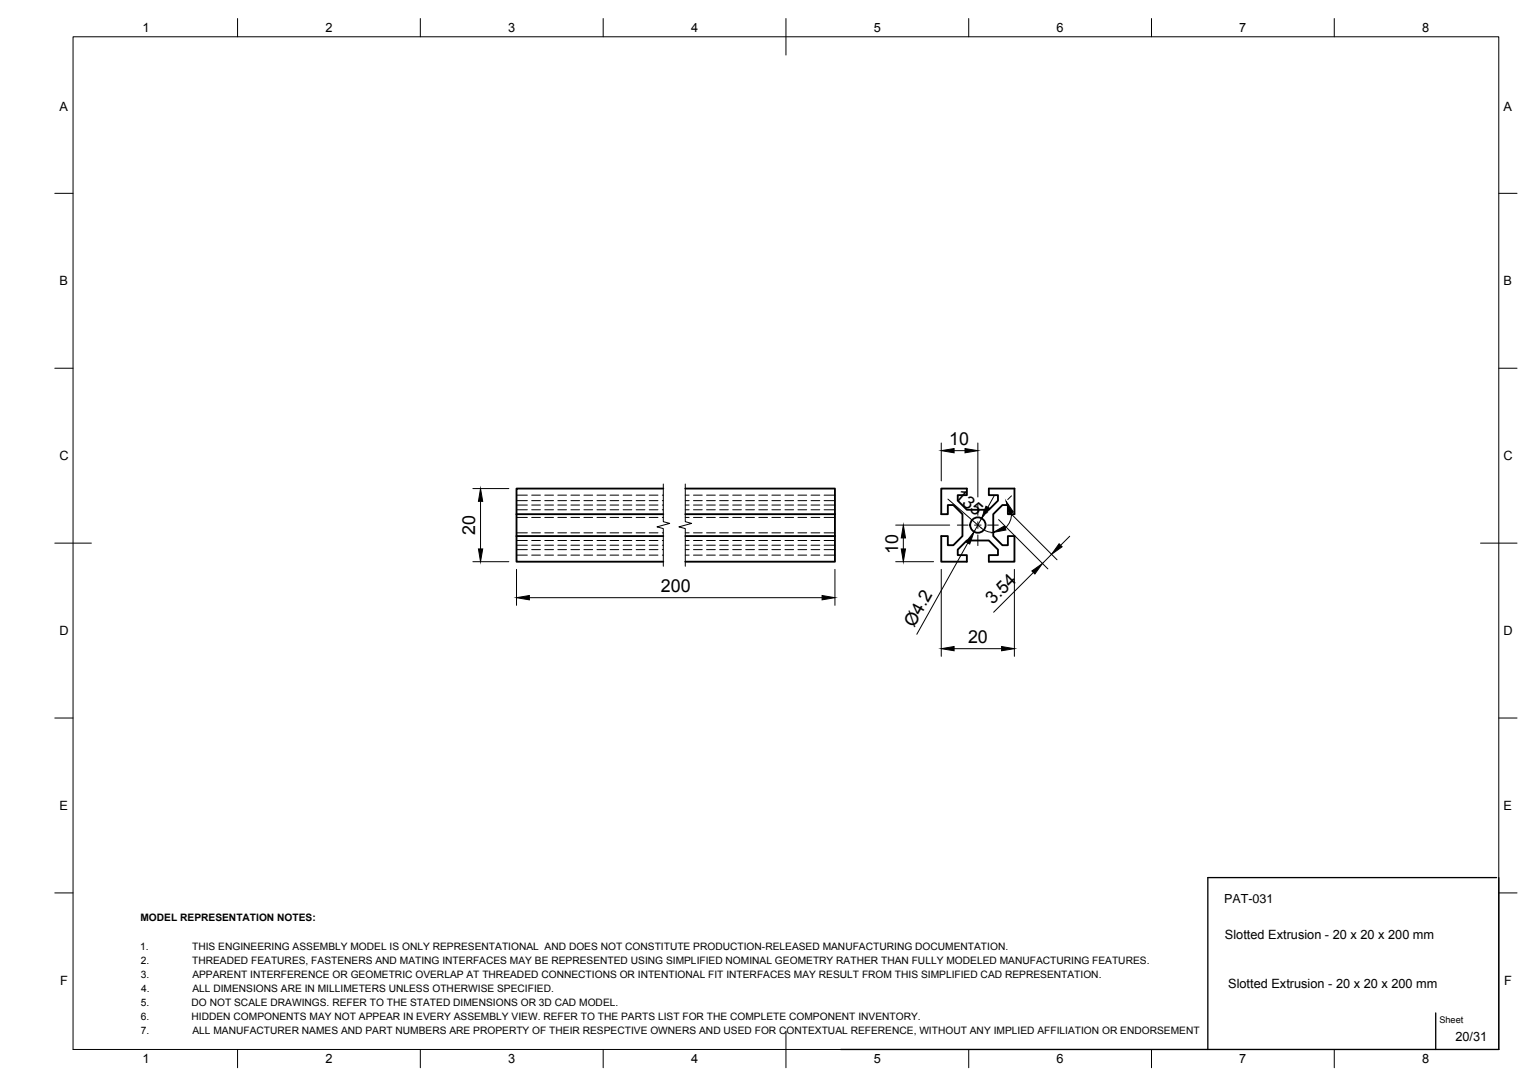
ISO-10303-21;
HEADER;
/* Generated by software containing ST-Developer
 * from STEP Tools, Inc. (www.steptools.com) 
 */

FILE_DESCRIPTION(
/* description */ ('Double-row support with tensioned shaft'),
/* implementation_level */ '2;1');

FILE_NAME(
/* name */ 'Slotted Extrusion - 20 x 20 x 200 mm.step',
/* time_stamp */ '2026-10-27T10:50:35-07:00',
/* author */ (''),
/* organization */ (''),
/* preprocessor_version */ 'ST-DEVELOPER v20.2',
/* originating_system */ 'Autodesk Translation Framework v15.17.0.0',
/* authorisation */ '');

FILE_SCHEMA (('AUTOMOTIVE_DESIGN { 1 0 10303 214 3 1 1 }'));
ENDSEC;

DATA;
#10=MECHANICAL_DESIGN_GEOMETRIC_PRESENTATION_REPRESENTATION('',(#494),#11559);
#430=SHAPE_REPRESENTATION_RELATIONSHIP('SRR','None',#11738,#462);
#462=ADVANCED_BREP_SHAPE_REPRESENTATION('',(#527),#11540);
#494=STYLED_ITEM('',(#11981),#527);
#527=MANIFOLD_SOLID_BREP('Body1',#6339);
#610=FACE_BOUND('',#1479,.T.);
#611=FACE_BOUND('',#1481,.T.);
#741=PLANE('',#6919);
#742=PLANE('',#6920);
#743=PLANE('',#6921);
#744=PLANE('',#6922);
#745=PLANE('',#6923);
#746=PLANE('',#6924);
#747=PLANE('',#6925);
#748=PLANE('',#6926);
#749=PLANE('',#6927);
#750=PLANE('',#6928);
#751=PLANE('',#6929);
#752=PLANE('',#6930);
#753=PLANE('',#6931);
#754=PLANE('',#6932);
#755=PLANE('',#6933);
#756=PLANE('',#6934);
#757=PLANE('',#6935);
#758=PLANE('',#6936);
#759=PLANE('',#6937);
#760=PLANE('',#6938);
#761=PLANE('',#6939);
#762=PLANE('',#6940);
#763=PLANE('',#6941);
#764=PLANE('',#6942);
#765=PLANE('',#6943);
#766=PLANE('',#6944);
#767=PLANE('',#6945);
#768=PLANE('',#6946);
#769=PLANE('',#6947);
#770=PLANE('',#6948);
#771=PLANE('',#6949);
#772=PLANE('',#6950);
#773=PLANE('',#6951);
#774=PLANE('',#6952);
#775=PLANE('',#6953);
#776=PLANE('',#6954);
#777=PLANE('',#6958);
#778=PLANE('',#6959);
#779=PLANE('',#6960);
#780=PLANE('',#6961);
#781=PLANE('',#6962);
#782=PLANE('',#6963);
#783=PLANE('',#6964);
#784=PLANE('',#6965);
#785=PLANE('',#6966);
#786=PLANE('',#6967);
#1021=FACE_OUTER_BOUND('',#1433,.T.);
#1022=FACE_OUTER_BOUND('',#1434,.T.);
#1023=FACE_OUTER_BOUND('',#1435,.T.);
#1024=FACE_OUTER_BOUND('',#1436,.T.);
#1025=FACE_OUTER_BOUND('',#1437,.T.);
#1026=FACE_OUTER_BOUND('',#1438,.T.);
#1027=FACE_OUTER_BOUND('',#1439,.T.);
#1028=FACE_OUTER_BOUND('',#1440,.T.);
#1029=FACE_OUTER_BOUND('',#1441,.T.);
#1030=FACE_OUTER_BOUND('',#1442,.T.);
#1031=FACE_OUTER_BOUND('',#1443,.T.);
#1032=FACE_OUTER_BOUND('',#1444,.T.);
#1033=FACE_OUTER_BOUND('',#1445,.T.);
#1034=FACE_OUTER_BOUND('',#1446,.T.);
#1035=FACE_OUTER_BOUND('',#1447,.T.);
#1036=FACE_OUTER_BOUND('',#1448,.T.);
#1037=FACE_OUTER_BOUND('',#1449,.T.);
#1038=FACE_OUTER_BOUND('',#1450,.T.);
#1039=FACE_OUTER_BOUND('',#1451,.T.);
#1040=FACE_OUTER_BOUND('',#1452,.T.);
#1041=FACE_OUTER_BOUND('',#1453,.T.);
#1042=FACE_OUTER_BOUND('',#1454,.T.);
#1043=FACE_OUTER_BOUND('',#1455,.T.);
#1044=FACE_OUTER_BOUND('',#1456,.T.);
#1045=FACE_OUTER_BOUND('',#1457,.T.);
#1046=FACE_OUTER_BOUND('',#1458,.T.);
#1047=FACE_OUTER_BOUND('',#1459,.T.);
#1048=FACE_OUTER_BOUND('',#1460,.T.);
#1049=FACE_OUTER_BOUND('',#1461,.T.);
#1050=FACE_OUTER_BOUND('',#1462,.T.);
#1051=FACE_OUTER_BOUND('',#1463,.T.);
#1052=FACE_OUTER_BOUND('',#1464,.T.);
#1053=FACE_OUTER_BOUND('',#1465,.T.);
#1054=FACE_OUTER_BOUND('',#1466,.T.);
#1055=FACE_OUTER_BOUND('',#1467,.T.);
#1056=FACE_OUTER_BOUND('',#1468,.T.);
#1057=FACE_OUTER_BOUND('',#1469,.T.);
#1058=FACE_OUTER_BOUND('',#1470,.T.);
#1059=FACE_OUTER_BOUND('',#1471,.T.);
#1060=FACE_OUTER_BOUND('',#1472,.T.);
#1061=FACE_OUTER_BOUND('',#1473,.T.);
#1062=FACE_OUTER_BOUND('',#1474,.T.);
#1063=FACE_OUTER_BOUND('',#1475,.T.);
#1064=FACE_OUTER_BOUND('',#1476,.T.);
#1065=FACE_OUTER_BOUND('',#1477,.T.);
#1066=FACE_OUTER_BOUND('',#1478,.T.);
#1067=FACE_OUTER_BOUND('',#1480,.T.);
#1433=EDGE_LOOP('',(#4774,#4775,#4776,#4777));
#1434=EDGE_LOOP('',(#4778,#4779,#4780,#4781));
#1435=EDGE_LOOP('',(#4782,#4783,#4784,#4785));
#1436=EDGE_LOOP('',(#4786,#4787,#4788,#4789));
#1437=EDGE_LOOP('',(#4790,#4791,#4792,#4793));
#1438=EDGE_LOOP('',(#4794,#4795,#4796,#4797));
#1439=EDGE_LOOP('',(#4798,#4799,#4800,#4801));
#1440=EDGE_LOOP('',(#4802,#4803,#4804,#4805));
#1441=EDGE_LOOP('',(#4806,#4807,#4808,#4809));
#1442=EDGE_LOOP('',(#4810,#4811,#4812,#4813));
#1443=EDGE_LOOP('',(#4814,#4815,#4816,#4817));
#1444=EDGE_LOOP('',(#4818,#4819,#4820,#4821));
#1445=EDGE_LOOP('',(#4822,#4823,#4824,#4825));
#1446=EDGE_LOOP('',(#4826,#4827,#4828,#4829));
#1447=EDGE_LOOP('',(#4830,#4831,#4832,#4833));
#1448=EDGE_LOOP('',(#4834,#4835,#4836,#4837));
#1449=EDGE_LOOP('',(#4838,#4839,#4840,#4841));
#1450=EDGE_LOOP('',(#4842,#4843,#4844,#4845));
#1451=EDGE_LOOP('',(#4846,#4847,#4848,#4849));
#1452=EDGE_LOOP('',(#4850,#4851,#4852,#4853));
#1453=EDGE_LOOP('',(#4854,#4855,#4856,#4857));
#1454=EDGE_LOOP('',(#4858,#4859,#4860,#4861));
#1455=EDGE_LOOP('',(#4862,#4863,#4864,#4865));
#1456=EDGE_LOOP('',(#4866,#4867,#4868,#4869));
#1457=EDGE_LOOP('',(#4870,#4871,#4872,#4873));
#1458=EDGE_LOOP('',(#4874,#4875,#4876,#4877));
#1459=EDGE_LOOP('',(#4878,#4879,#4880,#4881));
#1460=EDGE_LOOP('',(#4882,#4883,#4884,#4885));
#1461=EDGE_LOOP('',(#4886,#4887,#4888,#4889));
#1462=EDGE_LOOP('',(#4890,#4891,#4892,#4893));
#1463=EDGE_LOOP('',(#4894,#4895,#4896,#4897));
#1464=EDGE_LOOP('',(#4898,#4899,#4900,#4901));
#1465=EDGE_LOOP('',(#4902,#4903,#4904,#4905));
#1466=EDGE_LOOP('',(#4906,#4907,#4908,#4909));
#1467=EDGE_LOOP('',(#4910,#4911,#4912,#4913));
#1468=EDGE_LOOP('',(#4914,#4915,#4916,#4917));
#1469=EDGE_LOOP('',(#4918,#4919,#4920,#4921));
#1470=EDGE_LOOP('',(#4922,#4923,#4924,#4925));
#1471=EDGE_LOOP('',(#4926,#4927,#4928,#4929));
#1472=EDGE_LOOP('',(#4930,#4931,#4932,#4933));
#1473=EDGE_LOOP('',(#4934,#4935,#4936,#4937));
#1474=EDGE_LOOP('',(#4938,#4939,#4940,#4941));
#1475=EDGE_LOOP('',(#4942,#4943,#4944,#4945));
#1476=EDGE_LOOP('',(#4946,#4947,#4948,#4949));
#1477=EDGE_LOOP('',(#4950,#4951,#4952,#4953));
#1478=EDGE_LOOP('',(#4954,#4955,#4956,#4957,#4958,#4959,#4960,#4961,#4962,
#4963,#4964,#4965,#4966,#4967,#4968,#4969,#4970,#4971,#4972,#4973,#4974,
#4975,#4976,#4977,#4978,#4979,#4980,#4981,#4982,#4983,#4984,#4985,#4986,
#4987,#4988,#4989,#4990,#4991,#4992,#4993,#4994,#4995,#4996,#4997));
#1479=EDGE_LOOP('',(#4998));
#1480=EDGE_LOOP('',(#4999,#5000,#5001,#5002,#5003,#5004,#5005,#5006,#5007,
#5008,#5009,#5010,#5011,#5012,#5013,#5014,#5015,#5016,#5017,#5018,#5019,
#5020,#5021,#5022,#5023,#5024,#5025,#5026,#5027,#5028,#5029,#5030,#5031,
#5032,#5033,#5034,#5035,#5036,#5037,#5038,#5039,#5040,#5041,#5042));
#1481=EDGE_LOOP('',(#5043));
#1880=LINE('',#9729,#2427);
#1881=LINE('',#9731,#2428);
#1882=LINE('',#9733,#2429);
#1883=LINE('',#9734,#2430);
#1884=LINE('',#9737,#2431);
#1885=LINE('',#9739,#2432);
#1886=LINE('',#9740,#2433);
#1887=LINE('',#9743,#2434);
#1888=LINE('',#9745,#2435);
#1889=LINE('',#9746,#2436);
#1890=LINE('',#9749,#2437);
#1891=LINE('',#9751,#2438);
#1892=LINE('',#9752,#2439);
#1893=LINE('',#9755,#2440);
#1894=LINE('',#9757,#2441);
#1895=LINE('',#9758,#2442);
#1896=LINE('',#9761,#2443);
#1897=LINE('',#9763,#2444);
#1898=LINE('',#9764,#2445);
#1899=LINE('',#9767,#2446);
#1900=LINE('',#9769,#2447);
#1901=LINE('',#9770,#2448);
#1902=LINE('',#9773,#2449);
#1903=LINE('',#9775,#2450);
#1904=LINE('',#9776,#2451);
#1905=LINE('',#9779,#2452);
#1906=LINE('',#9781,#2453);
#1907=LINE('',#9782,#2454);
#1908=LINE('',#9786,#2455);
#1909=LINE('',#9788,#2456);
#1910=LINE('',#9790,#2457);
#1911=LINE('',#9791,#2458);
#1912=LINE('',#9794,#2459);
#1913=LINE('',#9796,#2460);
#1914=LINE('',#9797,#2461);
#1915=LINE('',#9800,#2462);
#1916=LINE('',#9802,#2463);
#1917=LINE('',#9803,#2464);
#1918=LINE('',#9806,#2465);
#1919=LINE('',#9808,#2466);
#1920=LINE('',#9809,#2467);
#1921=LINE('',#9812,#2468);
#1922=LINE('',#9814,#2469);
#1923=LINE('',#9815,#2470);
#1924=LINE('',#9818,#2471);
#1925=LINE('',#9820,#2472);
#1926=LINE('',#9821,#2473);
#1927=LINE('',#9824,#2474);
#1928=LINE('',#9826,#2475);
#1929=LINE('',#9827,#2476);
#1930=LINE('',#9830,#2477);
#1931=LINE('',#9832,#2478);
#1932=LINE('',#9833,#2479);
#1933=LINE('',#9836,#2480);
#1934=LINE('',#9838,#2481);
#1935=LINE('',#9839,#2482);
#1936=LINE('',#9843,#2483);
#1937=LINE('',#9845,#2484);
#1938=LINE('',#9847,#2485);
#1939=LINE('',#9848,#2486);
#1940=LINE('',#9851,#2487);
#1941=LINE('',#9853,#2488);
#1942=LINE('',#9854,#2489);
#1943=LINE('',#9857,#2490);
#1944=LINE('',#9859,#2491);
#1945=LINE('',#9860,#2492);
#1946=LINE('',#9863,#2493);
#1947=LINE('',#9865,#2494);
#1948=LINE('',#9866,#2495);
#1949=LINE('',#9869,#2496);
#1950=LINE('',#9871,#2497);
#1951=LINE('',#9872,#2498);
#1952=LINE('',#9875,#2499);
#1953=LINE('',#9877,#2500);
#1954=LINE('',#9878,#2501);
#1955=LINE('',#9881,#2502);
#1956=LINE('',#9883,#2503);
#1957=LINE('',#9884,#2504);
#1958=LINE('',#9887,#2505);
#1959=LINE('',#9889,#2506);
#1960=LINE('',#9890,#2507);
#1961=LINE('',#9893,#2508);
#1962=LINE('',#9895,#2509);
#1963=LINE('',#9896,#2510);
#1964=LINE('',#9900,#2511);
#1965=LINE('',#9902,#2512);
#1966=LINE('',#9904,#2513);
#1967=LINE('',#9905,#2514);
#1968=LINE('',#9908,#2515);
#1969=LINE('',#9910,#2516);
#1970=LINE('',#9911,#2517);
#1971=LINE('',#9914,#2518);
#1972=LINE('',#9916,#2519);
#1973=LINE('',#9917,#2520);
#1974=LINE('',#9920,#2521);
#1975=LINE('',#9922,#2522);
#1976=LINE('',#9923,#2523);
#1977=LINE('',#9926,#2524);
#1978=LINE('',#9928,#2525);
#1979=LINE('',#9929,#2526);
#1980=LINE('',#9932,#2527);
#1981=LINE('',#9934,#2528);
#1982=LINE('',#9935,#2529);
#1983=LINE('',#9938,#2530);
#1984=LINE('',#9940,#2531);
#1985=LINE('',#9941,#2532);
#1986=LINE('',#9944,#2533);
#1987=LINE('',#9946,#2534);
#1988=LINE('',#9947,#2535);
#1989=LINE('',#9950,#2536);
#1990=LINE('',#9952,#2537);
#1991=LINE('',#9953,#2538);
#1992=LINE('',#9958,#2539);
#1993=LINE('',#9962,#2540);
#1994=LINE('',#9964,#2541);
#1995=LINE('',#9965,#2542);
#1996=LINE('',#9968,#2543);
#1997=LINE('',#9970,#2544);
#1998=LINE('',#9971,#2545);
#1999=LINE('',#9973,#2546);
#2000=LINE('',#9974,#2547);
#2001=LINE('',#9977,#2548);
#2002=LINE('',#9979,#2549);
#2003=LINE('',#9980,#2550);
#2004=LINE('',#9982,#2551);
#2005=LINE('',#9983,#2552);
#2006=LINE('',#9986,#2553);
#2007=LINE('',#9988,#2554);
#2008=LINE('',#9989,#2555);
#2009=LINE('',#9991,#2556);
#2010=LINE('',#9992,#2557);
#2011=LINE('',#9994,#2558);
#2012=LINE('',#9995,#2559);
#2427=VECTOR('',#7923,1.);
#2428=VECTOR('',#7924,1.);
#2429=VECTOR('',#7925,1.);
#2430=VECTOR('',#7926,1.);
#2431=VECTOR('',#7929,1.);
#2432=VECTOR('',#7930,1.);
#2433=VECTOR('',#7931,1.);
#2434=VECTOR('',#7934,1.);
#2435=VECTOR('',#7935,1.);
#2436=VECTOR('',#7936,1.);
#2437=VECTOR('',#7939,1.);
#2438=VECTOR('',#7940,1.);
#2439=VECTOR('',#7941,1.);
#2440=VECTOR('',#7944,1.);
#2441=VECTOR('',#7945,1.);
#2442=VECTOR('',#7946,1.);
#2443=VECTOR('',#7949,1.);
#2444=VECTOR('',#7950,1.);
#2445=VECTOR('',#7951,1.);
#2446=VECTOR('',#7954,1.);
#2447=VECTOR('',#7955,1.);
#2448=VECTOR('',#7956,1.);
#2449=VECTOR('',#7959,1.);
#2450=VECTOR('',#7960,1.);
#2451=VECTOR('',#7961,1.);
#2452=VECTOR('',#7964,1.);
#2453=VECTOR('',#7965,1.);
#2454=VECTOR('',#7966,1.);
#2455=VECTOR('',#7969,1.);
#2456=VECTOR('',#7970,1.);
#2457=VECTOR('',#7971,1.);
#2458=VECTOR('',#7972,1.);
#2459=VECTOR('',#7975,1.);
#2460=VECTOR('',#7976,1.);
#2461=VECTOR('',#7977,1.);
#2462=VECTOR('',#7980,1.);
#2463=VECTOR('',#7981,1.);
#2464=VECTOR('',#7982,1.);
#2465=VECTOR('',#7985,1.);
#2466=VECTOR('',#7986,1.);
#2467=VECTOR('',#7987,1.);
#2468=VECTOR('',#7990,1.);
#2469=VECTOR('',#7991,1.);
#2470=VECTOR('',#7992,1.);
#2471=VECTOR('',#7995,1.);
#2472=VECTOR('',#7996,1.);
#2473=VECTOR('',#7997,1.);
#2474=VECTOR('',#8000,1.);
#2475=VECTOR('',#8001,1.);
#2476=VECTOR('',#8002,1.);
#2477=VECTOR('',#8005,1.);
#2478=VECTOR('',#8006,1.);
#2479=VECTOR('',#8007,1.);
#2480=VECTOR('',#8010,1.);
#2481=VECTOR('',#8011,1.);
#2482=VECTOR('',#8012,1.);
#2483=VECTOR('',#8015,1.);
#2484=VECTOR('',#8016,1.);
#2485=VECTOR('',#8017,1.);
#2486=VECTOR('',#8018,1.);
#2487=VECTOR('',#8021,1.);
#2488=VECTOR('',#8022,1.);
#2489=VECTOR('',#8023,1.);
#2490=VECTOR('',#8026,1.);
#2491=VECTOR('',#8027,1.);
#2492=VECTOR('',#8028,1.);
#2493=VECTOR('',#8031,1.);
#2494=VECTOR('',#8032,1.);
#2495=VECTOR('',#8033,1.);
#2496=VECTOR('',#8036,1.);
#2497=VECTOR('',#8037,1.);
#2498=VECTOR('',#8038,1.);
#2499=VECTOR('',#8041,1.);
#2500=VECTOR('',#8042,1.);
#2501=VECTOR('',#8043,1.);
#2502=VECTOR('',#8046,1.);
#2503=VECTOR('',#8047,1.);
#2504=VECTOR('',#8048,1.);
#2505=VECTOR('',#8051,1.);
#2506=VECTOR('',#8052,1.);
#2507=VECTOR('',#8053,1.);
#2508=VECTOR('',#8056,1.);
#2509=VECTOR('',#8057,1.);
#2510=VECTOR('',#8058,1.);
#2511=VECTOR('',#8061,1.);
#2512=VECTOR('',#8062,1.);
#2513=VECTOR('',#8063,1.);
#2514=VECTOR('',#8064,1.);
#2515=VECTOR('',#8067,1.);
#2516=VECTOR('',#8068,1.);
#2517=VECTOR('',#8069,1.);
#2518=VECTOR('',#8072,1.);
#2519=VECTOR('',#8073,1.);
#2520=VECTOR('',#8074,1.);
#2521=VECTOR('',#8077,1.);
#2522=VECTOR('',#8078,1.);
#2523=VECTOR('',#8079,1.);
#2524=VECTOR('',#8082,1.);
#2525=VECTOR('',#8083,1.);
#2526=VECTOR('',#8084,1.);
#2527=VECTOR('',#8087,1.);
#2528=VECTOR('',#8088,1.);
#2529=VECTOR('',#8089,1.);
#2530=VECTOR('',#8092,1.);
#2531=VECTOR('',#8093,1.);
#2532=VECTOR('',#8094,1.);
#2533=VECTOR('',#8097,1.);
#2534=VECTOR('',#8098,1.);
#2535=VECTOR('',#8099,1.);
#2536=VECTOR('',#8102,1.);
#2537=VECTOR('',#8103,1.);
#2538=VECTOR('',#8104,1.);
#2539=VECTOR('',#8109,0.21);
#2540=VECTOR('',#8114,1.);
#2541=VECTOR('',#8115,1.);
#2542=VECTOR('',#8116,1.);
#2543=VECTOR('',#8119,1.);
#2544=VECTOR('',#8120,1.);
#2545=VECTOR('',#8121,1.);
#2546=VECTOR('',#8124,1.);
#2547=VECTOR('',#8125,1.);
#2548=VECTOR('',#8128,1.);
#2549=VECTOR('',#8129,1.);
#2550=VECTOR('',#8130,1.);
#2551=VECTOR('',#8133,1.);
#2552=VECTOR('',#8134,1.);
#2553=VECTOR('',#8137,1.);
#2554=VECTOR('',#8138,1.);
#2555=VECTOR('',#8139,1.);
#2556=VECTOR('',#8142,1.);
#2557=VECTOR('',#8143,1.);
#2558=VECTOR('',#8146,1.);
#2559=VECTOR('',#8147,1.);
#2920=CIRCLE('',#6956,0.21);
#2921=CIRCLE('',#6957,0.21);
#3175=VERTEX_POINT('',#9727);
#3176=VERTEX_POINT('',#9728);
#3177=VERTEX_POINT('',#9730);
#3178=VERTEX_POINT('',#9732);
#3179=VERTEX_POINT('',#9736);
#3180=VERTEX_POINT('',#9738);
#3181=VERTEX_POINT('',#9742);
#3182=VERTEX_POINT('',#9744);
#3183=VERTEX_POINT('',#9748);
#3184=VERTEX_POINT('',#9750);
#3185=VERTEX_POINT('',#9754);
#3186=VERTEX_POINT('',#9756);
#3187=VERTEX_POINT('',#9760);
#3188=VERTEX_POINT('',#9762);
#3189=VERTEX_POINT('',#9766);
#3190=VERTEX_POINT('',#9768);
#3191=VERTEX_POINT('',#9772);
#3192=VERTEX_POINT('',#9774);
#3193=VERTEX_POINT('',#9778);
#3194=VERTEX_POINT('',#9780);
#3195=VERTEX_POINT('',#9784);
#3196=VERTEX_POINT('',#9785);
#3197=VERTEX_POINT('',#9787);
#3198=VERTEX_POINT('',#9789);
#3199=VERTEX_POINT('',#9793);
#3200=VERTEX_POINT('',#9795);
#3201=VERTEX_POINT('',#9799);
#3202=VERTEX_POINT('',#9801);
#3203=VERTEX_POINT('',#9805);
#3204=VERTEX_POINT('',#9807);
#3205=VERTEX_POINT('',#9811);
#3206=VERTEX_POINT('',#9813);
#3207=VERTEX_POINT('',#9817);
#3208=VERTEX_POINT('',#9819);
#3209=VERTEX_POINT('',#9823);
#3210=VERTEX_POINT('',#9825);
#3211=VERTEX_POINT('',#9829);
#3212=VERTEX_POINT('',#9831);
#3213=VERTEX_POINT('',#9835);
#3214=VERTEX_POINT('',#9837);
#3215=VERTEX_POINT('',#9841);
#3216=VERTEX_POINT('',#9842);
#3217=VERTEX_POINT('',#9844);
#3218=VERTEX_POINT('',#9846);
#3219=VERTEX_POINT('',#9850);
#3220=VERTEX_POINT('',#9852);
#3221=VERTEX_POINT('',#9856);
#3222=VERTEX_POINT('',#9858);
#3223=VERTEX_POINT('',#9862);
#3224=VERTEX_POINT('',#9864);
#3225=VERTEX_POINT('',#9868);
#3226=VERTEX_POINT('',#9870);
#3227=VERTEX_POINT('',#9874);
#3228=VERTEX_POINT('',#9876);
#3229=VERTEX_POINT('',#9880);
#3230=VERTEX_POINT('',#9882);
#3231=VERTEX_POINT('',#9886);
#3232=VERTEX_POINT('',#9888);
#3233=VERTEX_POINT('',#9892);
#3234=VERTEX_POINT('',#9894);
#3235=VERTEX_POINT('',#9898);
#3236=VERTEX_POINT('',#9899);
#3237=VERTEX_POINT('',#9901);
#3238=VERTEX_POINT('',#9903);
#3239=VERTEX_POINT('',#9907);
#3240=VERTEX_POINT('',#9909);
#3241=VERTEX_POINT('',#9913);
#3242=VERTEX_POINT('',#9915);
#3243=VERTEX_POINT('',#9919);
#3244=VERTEX_POINT('',#9921);
#3245=VERTEX_POINT('',#9925);
#3246=VERTEX_POINT('',#9927);
#3247=VERTEX_POINT('',#9931);
#3248=VERTEX_POINT('',#9933);
#3249=VERTEX_POINT('',#9937);
#3250=VERTEX_POINT('',#9939);
#3251=VERTEX_POINT('',#9943);
#3252=VERTEX_POINT('',#9945);
#3253=VERTEX_POINT('',#9949);
#3254=VERTEX_POINT('',#9951);
#3255=VERTEX_POINT('',#9955);
#3256=VERTEX_POINT('',#9957);
#3257=VERTEX_POINT('',#9961);
#3258=VERTEX_POINT('',#9963);
#3259=VERTEX_POINT('',#9967);
#3260=VERTEX_POINT('',#9969);
#3261=VERTEX_POINT('',#9976);
#3262=VERTEX_POINT('',#9978);
#3263=VERTEX_POINT('',#9985);
#3264=VERTEX_POINT('',#9987);
#3772=EDGE_CURVE('',#3175,#3176,#1880,.T.);
#3773=EDGE_CURVE('',#3175,#3177,#1881,.T.);
#3774=EDGE_CURVE('',#3178,#3177,#1882,.T.);
#3775=EDGE_CURVE('',#3176,#3178,#1883,.T.);
#3776=EDGE_CURVE('',#3179,#3175,#1884,.T.);
#3777=EDGE_CURVE('',#3179,#3180,#1885,.T.);
#3778=EDGE_CURVE('',#3177,#3180,#1886,.T.);
#3779=EDGE_CURVE('',#3181,#3179,#1887,.T.);
#3780=EDGE_CURVE('',#3181,#3182,#1888,.T.);
#3781=EDGE_CURVE('',#3180,#3182,#1889,.T.);
#3782=EDGE_CURVE('',#3183,#3181,#1890,.T.);
#3783=EDGE_CURVE('',#3183,#3184,#1891,.T.);
#3784=EDGE_CURVE('',#3182,#3184,#1892,.T.);
#3785=EDGE_CURVE('',#3185,#3183,#1893,.T.);
#3786=EDGE_CURVE('',#3185,#3186,#1894,.T.);
#3787=EDGE_CURVE('',#3184,#3186,#1895,.T.);
#3788=EDGE_CURVE('',#3187,#3185,#1896,.T.);
#3789=EDGE_CURVE('',#3187,#3188,#1897,.T.);
#3790=EDGE_CURVE('',#3186,#3188,#1898,.T.);
#3791=EDGE_CURVE('',#3189,#3187,#1899,.T.);
#3792=EDGE_CURVE('',#3189,#3190,#1900,.T.);
#3793=EDGE_CURVE('',#3188,#3190,#1901,.T.);
#3794=EDGE_CURVE('',#3191,#3189,#1902,.T.);
#3795=EDGE_CURVE('',#3191,#3192,#1903,.T.);
#3796=EDGE_CURVE('',#3190,#3192,#1904,.T.);
#3797=EDGE_CURVE('',#3193,#3191,#1905,.T.);
#3798=EDGE_CURVE('',#3194,#3193,#1906,.T.);
#3799=EDGE_CURVE('',#3192,#3194,#1907,.T.);
#3800=EDGE_CURVE('',#3195,#3196,#1908,.T.);
#3801=EDGE_CURVE('',#3195,#3197,#1909,.T.);
#3802=EDGE_CURVE('',#3198,#3197,#1910,.T.);
#3803=EDGE_CURVE('',#3196,#3198,#1911,.T.);
#3804=EDGE_CURVE('',#3199,#3195,#1912,.T.);
#3805=EDGE_CURVE('',#3199,#3200,#1913,.T.);
#3806=EDGE_CURVE('',#3197,#3200,#1914,.T.);
#3807=EDGE_CURVE('',#3201,#3199,#1915,.T.);
#3808=EDGE_CURVE('',#3201,#3202,#1916,.T.);
#3809=EDGE_CURVE('',#3200,#3202,#1917,.T.);
#3810=EDGE_CURVE('',#3203,#3201,#1918,.T.);
#3811=EDGE_CURVE('',#3203,#3204,#1919,.T.);
#3812=EDGE_CURVE('',#3202,#3204,#1920,.T.);
#3813=EDGE_CURVE('',#3205,#3203,#1921,.T.);
#3814=EDGE_CURVE('',#3205,#3206,#1922,.T.);
#3815=EDGE_CURVE('',#3204,#3206,#1923,.T.);
#3816=EDGE_CURVE('',#3207,#3205,#1924,.T.);
#3817=EDGE_CURVE('',#3207,#3208,#1925,.T.);
#3818=EDGE_CURVE('',#3206,#3208,#1926,.T.);
#3819=EDGE_CURVE('',#3209,#3207,#1927,.T.);
#3820=EDGE_CURVE('',#3209,#3210,#1928,.T.);
#3821=EDGE_CURVE('',#3208,#3210,#1929,.T.);
#3822=EDGE_CURVE('',#3211,#3209,#1930,.T.);
#3823=EDGE_CURVE('',#3211,#3212,#1931,.T.);
#3824=EDGE_CURVE('',#3210,#3212,#1932,.T.);
#3825=EDGE_CURVE('',#3213,#3211,#1933,.T.);
#3826=EDGE_CURVE('',#3214,#3213,#1934,.T.);
#3827=EDGE_CURVE('',#3212,#3214,#1935,.T.);
#3828=EDGE_CURVE('',#3215,#3216,#1936,.T.);
#3829=EDGE_CURVE('',#3215,#3217,#1937,.T.);
#3830=EDGE_CURVE('',#3218,#3217,#1938,.T.);
#3831=EDGE_CURVE('',#3216,#3218,#1939,.T.);
#3832=EDGE_CURVE('',#3219,#3215,#1940,.T.);
#3833=EDGE_CURVE('',#3219,#3220,#1941,.T.);
#3834=EDGE_CURVE('',#3217,#3220,#1942,.T.);
#3835=EDGE_CURVE('',#3221,#3219,#1943,.T.);
#3836=EDGE_CURVE('',#3221,#3222,#1944,.T.);
#3837=EDGE_CURVE('',#3220,#3222,#1945,.T.);
#3838=EDGE_CURVE('',#3223,#3221,#1946,.T.);
#3839=EDGE_CURVE('',#3223,#3224,#1947,.T.);
#3840=EDGE_CURVE('',#3222,#3224,#1948,.T.);
#3841=EDGE_CURVE('',#3225,#3223,#1949,.T.);
#3842=EDGE_CURVE('',#3225,#3226,#1950,.T.);
#3843=EDGE_CURVE('',#3224,#3226,#1951,.T.);
#3844=EDGE_CURVE('',#3227,#3225,#1952,.T.);
#3845=EDGE_CURVE('',#3227,#3228,#1953,.T.);
#3846=EDGE_CURVE('',#3226,#3228,#1954,.T.);
#3847=EDGE_CURVE('',#3229,#3227,#1955,.T.);
#3848=EDGE_CURVE('',#3229,#3230,#1956,.T.);
#3849=EDGE_CURVE('',#3228,#3230,#1957,.T.);
#3850=EDGE_CURVE('',#3231,#3229,#1958,.T.);
#3851=EDGE_CURVE('',#3231,#3232,#1959,.T.);
#3852=EDGE_CURVE('',#3230,#3232,#1960,.T.);
#3853=EDGE_CURVE('',#3233,#3231,#1961,.T.);
#3854=EDGE_CURVE('',#3234,#3233,#1962,.T.);
#3855=EDGE_CURVE('',#3232,#3234,#1963,.T.);
#3856=EDGE_CURVE('',#3235,#3236,#1964,.T.);
#3857=EDGE_CURVE('',#3235,#3237,#1965,.T.);
#3858=EDGE_CURVE('',#3238,#3237,#1966,.T.);
#3859=EDGE_CURVE('',#3236,#3238,#1967,.T.);
#3860=EDGE_CURVE('',#3239,#3235,#1968,.T.);
#3861=EDGE_CURVE('',#3239,#3240,#1969,.T.);
#3862=EDGE_CURVE('',#3237,#3240,#1970,.T.);
#3863=EDGE_CURVE('',#3241,#3239,#1971,.T.);
#3864=EDGE_CURVE('',#3241,#3242,#1972,.T.);
#3865=EDGE_CURVE('',#3240,#3242,#1973,.T.);
#3866=EDGE_CURVE('',#3243,#3241,#1974,.T.);
#3867=EDGE_CURVE('',#3243,#3244,#1975,.T.);
#3868=EDGE_CURVE('',#3242,#3244,#1976,.T.);
#3869=EDGE_CURVE('',#3245,#3243,#1977,.T.);
#3870=EDGE_CURVE('',#3245,#3246,#1978,.T.);
#3871=EDGE_CURVE('',#3244,#3246,#1979,.T.);
#3872=EDGE_CURVE('',#3247,#3245,#1980,.T.);
#3873=EDGE_CURVE('',#3247,#3248,#1981,.T.);
#3874=EDGE_CURVE('',#3246,#3248,#1982,.T.);
#3875=EDGE_CURVE('',#3249,#3247,#1983,.T.);
#3876=EDGE_CURVE('',#3249,#3250,#1984,.T.);
#3877=EDGE_CURVE('',#3248,#3250,#1985,.T.);
#3878=EDGE_CURVE('',#3251,#3249,#1986,.T.);
#3879=EDGE_CURVE('',#3251,#3252,#1987,.T.);
#3880=EDGE_CURVE('',#3250,#3252,#1988,.T.);
#3881=EDGE_CURVE('',#3253,#3251,#1989,.T.);
#3882=EDGE_CURVE('',#3254,#3253,#1990,.T.);
#3883=EDGE_CURVE('',#3252,#3254,#1991,.T.);
#3884=EDGE_CURVE('',#3255,#3255,#2920,.T.);
#3885=EDGE_CURVE('',#3255,#3256,#1992,.T.);
#3886=EDGE_CURVE('',#3256,#3256,#2921,.T.);
#3887=EDGE_CURVE('',#3193,#3257,#1993,.T.);
#3888=EDGE_CURVE('',#3257,#3258,#1994,.T.);
#3889=EDGE_CURVE('',#3194,#3258,#1995,.T.);
#3890=EDGE_CURVE('',#3259,#3178,#1996,.T.);
#3891=EDGE_CURVE('',#3260,#3259,#1997,.T.);
#3892=EDGE_CURVE('',#3260,#3176,#1998,.T.);
#3893=EDGE_CURVE('',#3213,#3260,#1999,.T.);
#3894=EDGE_CURVE('',#3214,#3259,#2000,.T.);
#3895=EDGE_CURVE('',#3261,#3198,#2001,.T.);
#3896=EDGE_CURVE('',#3262,#3261,#2002,.T.);
#3897=EDGE_CURVE('',#3262,#3196,#2003,.T.);
#3898=EDGE_CURVE('',#3233,#3262,#2004,.T.);
#3899=EDGE_CURVE('',#3234,#3261,#2005,.T.);
#3900=EDGE_CURVE('',#3263,#3218,#2006,.T.);
#3901=EDGE_CURVE('',#3264,#3263,#2007,.T.);
#3902=EDGE_CURVE('',#3264,#3216,#2008,.T.);
#3903=EDGE_CURVE('',#3253,#3264,#2009,.T.);
#3904=EDGE_CURVE('',#3254,#3263,#2010,.T.);
#3905=EDGE_CURVE('',#3258,#3238,#2011,.T.);
#3906=EDGE_CURVE('',#3257,#3236,#2012,.T.);
#4774=ORIENTED_EDGE('',*,*,#3772,.F.);
#4775=ORIENTED_EDGE('',*,*,#3773,.T.);
#4776=ORIENTED_EDGE('',*,*,#3774,.F.);
#4777=ORIENTED_EDGE('',*,*,#3775,.F.);
#4778=ORIENTED_EDGE('',*,*,#3776,.F.);
#4779=ORIENTED_EDGE('',*,*,#3777,.T.);
#4780=ORIENTED_EDGE('',*,*,#3778,.F.);
#4781=ORIENTED_EDGE('',*,*,#3773,.F.);
#4782=ORIENTED_EDGE('',*,*,#3779,.F.);
#4783=ORIENTED_EDGE('',*,*,#3780,.T.);
#4784=ORIENTED_EDGE('',*,*,#3781,.F.);
#4785=ORIENTED_EDGE('',*,*,#3777,.F.);
#4786=ORIENTED_EDGE('',*,*,#3782,.F.);
#4787=ORIENTED_EDGE('',*,*,#3783,.T.);
#4788=ORIENTED_EDGE('',*,*,#3784,.F.);
#4789=ORIENTED_EDGE('',*,*,#3780,.F.);
#4790=ORIENTED_EDGE('',*,*,#3785,.F.);
#4791=ORIENTED_EDGE('',*,*,#3786,.T.);
#4792=ORIENTED_EDGE('',*,*,#3787,.F.);
#4793=ORIENTED_EDGE('',*,*,#3783,.F.);
#4794=ORIENTED_EDGE('',*,*,#3788,.F.);
#4795=ORIENTED_EDGE('',*,*,#3789,.T.);
#4796=ORIENTED_EDGE('',*,*,#3790,.F.);
#4797=ORIENTED_EDGE('',*,*,#3786,.F.);
#4798=ORIENTED_EDGE('',*,*,#3791,.F.);
#4799=ORIENTED_EDGE('',*,*,#3792,.T.);
#4800=ORIENTED_EDGE('',*,*,#3793,.F.);
#4801=ORIENTED_EDGE('',*,*,#3789,.F.);
#4802=ORIENTED_EDGE('',*,*,#3794,.F.);
#4803=ORIENTED_EDGE('',*,*,#3795,.T.);
#4804=ORIENTED_EDGE('',*,*,#3796,.F.);
#4805=ORIENTED_EDGE('',*,*,#3792,.F.);
#4806=ORIENTED_EDGE('',*,*,#3797,.F.);
#4807=ORIENTED_EDGE('',*,*,#3798,.F.);
#4808=ORIENTED_EDGE('',*,*,#3799,.F.);
#4809=ORIENTED_EDGE('',*,*,#3795,.F.);
#4810=ORIENTED_EDGE('',*,*,#3800,.F.);
#4811=ORIENTED_EDGE('',*,*,#3801,.T.);
#4812=ORIENTED_EDGE('',*,*,#3802,.F.);
#4813=ORIENTED_EDGE('',*,*,#3803,.F.);
#4814=ORIENTED_EDGE('',*,*,#3804,.F.);
#4815=ORIENTED_EDGE('',*,*,#3805,.T.);
#4816=ORIENTED_EDGE('',*,*,#3806,.F.);
#4817=ORIENTED_EDGE('',*,*,#3801,.F.);
#4818=ORIENTED_EDGE('',*,*,#3807,.F.);
#4819=ORIENTED_EDGE('',*,*,#3808,.T.);
#4820=ORIENTED_EDGE('',*,*,#3809,.F.);
#4821=ORIENTED_EDGE('',*,*,#3805,.F.);
#4822=ORIENTED_EDGE('',*,*,#3810,.F.);
#4823=ORIENTED_EDGE('',*,*,#3811,.T.);
#4824=ORIENTED_EDGE('',*,*,#3812,.F.);
#4825=ORIENTED_EDGE('',*,*,#3808,.F.);
#4826=ORIENTED_EDGE('',*,*,#3813,.F.);
#4827=ORIENTED_EDGE('',*,*,#3814,.T.);
#4828=ORIENTED_EDGE('',*,*,#3815,.F.);
#4829=ORIENTED_EDGE('',*,*,#3811,.F.);
#4830=ORIENTED_EDGE('',*,*,#3816,.F.);
#4831=ORIENTED_EDGE('',*,*,#3817,.T.);
#4832=ORIENTED_EDGE('',*,*,#3818,.F.);
#4833=ORIENTED_EDGE('',*,*,#3814,.F.);
#4834=ORIENTED_EDGE('',*,*,#3819,.F.);
#4835=ORIENTED_EDGE('',*,*,#3820,.T.);
#4836=ORIENTED_EDGE('',*,*,#3821,.F.);
#4837=ORIENTED_EDGE('',*,*,#3817,.F.);
#4838=ORIENTED_EDGE('',*,*,#3822,.F.);
#4839=ORIENTED_EDGE('',*,*,#3823,.T.);
#4840=ORIENTED_EDGE('',*,*,#3824,.F.);
#4841=ORIENTED_EDGE('',*,*,#3820,.F.);
#4842=ORIENTED_EDGE('',*,*,#3825,.F.);
#4843=ORIENTED_EDGE('',*,*,#3826,.F.);
#4844=ORIENTED_EDGE('',*,*,#3827,.F.);
#4845=ORIENTED_EDGE('',*,*,#3823,.F.);
#4846=ORIENTED_EDGE('',*,*,#3828,.F.);
#4847=ORIENTED_EDGE('',*,*,#3829,.T.);
#4848=ORIENTED_EDGE('',*,*,#3830,.F.);
#4849=ORIENTED_EDGE('',*,*,#3831,.F.);
#4850=ORIENTED_EDGE('',*,*,#3832,.F.);
#4851=ORIENTED_EDGE('',*,*,#3833,.T.);
#4852=ORIENTED_EDGE('',*,*,#3834,.F.);
#4853=ORIENTED_EDGE('',*,*,#3829,.F.);
#4854=ORIENTED_EDGE('',*,*,#3835,.F.);
#4855=ORIENTED_EDGE('',*,*,#3836,.T.);
#4856=ORIENTED_EDGE('',*,*,#3837,.F.);
#4857=ORIENTED_EDGE('',*,*,#3833,.F.);
#4858=ORIENTED_EDGE('',*,*,#3838,.F.);
#4859=ORIENTED_EDGE('',*,*,#3839,.T.);
#4860=ORIENTED_EDGE('',*,*,#3840,.F.);
#4861=ORIENTED_EDGE('',*,*,#3836,.F.);
#4862=ORIENTED_EDGE('',*,*,#3841,.F.);
#4863=ORIENTED_EDGE('',*,*,#3842,.T.);
#4864=ORIENTED_EDGE('',*,*,#3843,.F.);
#4865=ORIENTED_EDGE('',*,*,#3839,.F.);
#4866=ORIENTED_EDGE('',*,*,#3844,.F.);
#4867=ORIENTED_EDGE('',*,*,#3845,.T.);
#4868=ORIENTED_EDGE('',*,*,#3846,.F.);
#4869=ORIENTED_EDGE('',*,*,#3842,.F.);
#4870=ORIENTED_EDGE('',*,*,#3847,.F.);
#4871=ORIENTED_EDGE('',*,*,#3848,.T.);
#4872=ORIENTED_EDGE('',*,*,#3849,.F.);
#4873=ORIENTED_EDGE('',*,*,#3845,.F.);
#4874=ORIENTED_EDGE('',*,*,#3850,.F.);
#4875=ORIENTED_EDGE('',*,*,#3851,.T.);
#4876=ORIENTED_EDGE('',*,*,#3852,.F.);
#4877=ORIENTED_EDGE('',*,*,#3848,.F.);
#4878=ORIENTED_EDGE('',*,*,#3853,.F.);
#4879=ORIENTED_EDGE('',*,*,#3854,.F.);
#4880=ORIENTED_EDGE('',*,*,#3855,.F.);
#4881=ORIENTED_EDGE('',*,*,#3851,.F.);
#4882=ORIENTED_EDGE('',*,*,#3856,.F.);
#4883=ORIENTED_EDGE('',*,*,#3857,.T.);
#4884=ORIENTED_EDGE('',*,*,#3858,.F.);
#4885=ORIENTED_EDGE('',*,*,#3859,.F.);
#4886=ORIENTED_EDGE('',*,*,#3860,.F.);
#4887=ORIENTED_EDGE('',*,*,#3861,.T.);
#4888=ORIENTED_EDGE('',*,*,#3862,.F.);
#4889=ORIENTED_EDGE('',*,*,#3857,.F.);
#4890=ORIENTED_EDGE('',*,*,#3863,.F.);
#4891=ORIENTED_EDGE('',*,*,#3864,.T.);
#4892=ORIENTED_EDGE('',*,*,#3865,.F.);
#4893=ORIENTED_EDGE('',*,*,#3861,.F.);
#4894=ORIENTED_EDGE('',*,*,#3866,.F.);
#4895=ORIENTED_EDGE('',*,*,#3867,.T.);
#4896=ORIENTED_EDGE('',*,*,#3868,.F.);
#4897=ORIENTED_EDGE('',*,*,#3864,.F.);
#4898=ORIENTED_EDGE('',*,*,#3869,.F.);
#4899=ORIENTED_EDGE('',*,*,#3870,.T.);
#4900=ORIENTED_EDGE('',*,*,#3871,.F.);
#4901=ORIENTED_EDGE('',*,*,#3867,.F.);
#4902=ORIENTED_EDGE('',*,*,#3872,.F.);
#4903=ORIENTED_EDGE('',*,*,#3873,.T.);
#4904=ORIENTED_EDGE('',*,*,#3874,.F.);
#4905=ORIENTED_EDGE('',*,*,#3870,.F.);
#4906=ORIENTED_EDGE('',*,*,#3875,.F.);
#4907=ORIENTED_EDGE('',*,*,#3876,.T.);
#4908=ORIENTED_EDGE('',*,*,#3877,.F.);
#4909=ORIENTED_EDGE('',*,*,#3873,.F.);
#4910=ORIENTED_EDGE('',*,*,#3878,.F.);
#4911=ORIENTED_EDGE('',*,*,#3879,.T.);
#4912=ORIENTED_EDGE('',*,*,#3880,.F.);
#4913=ORIENTED_EDGE('',*,*,#3876,.F.);
#4914=ORIENTED_EDGE('',*,*,#3881,.F.);
#4915=ORIENTED_EDGE('',*,*,#3882,.F.);
#4916=ORIENTED_EDGE('',*,*,#3883,.F.);
#4917=ORIENTED_EDGE('',*,*,#3879,.F.);
#4918=ORIENTED_EDGE('',*,*,#3884,.F.);
#4919=ORIENTED_EDGE('',*,*,#3885,.T.);
#4920=ORIENTED_EDGE('',*,*,#3886,.F.);
#4921=ORIENTED_EDGE('',*,*,#3885,.F.);
#4922=ORIENTED_EDGE('',*,*,#3798,.T.);
#4923=ORIENTED_EDGE('',*,*,#3887,.T.);
#4924=ORIENTED_EDGE('',*,*,#3888,.T.);
#4925=ORIENTED_EDGE('',*,*,#3889,.F.);
#4926=ORIENTED_EDGE('',*,*,#3775,.T.);
#4927=ORIENTED_EDGE('',*,*,#3890,.F.);
#4928=ORIENTED_EDGE('',*,*,#3891,.F.);
#4929=ORIENTED_EDGE('',*,*,#3892,.T.);
#4930=ORIENTED_EDGE('',*,*,#3826,.T.);
#4931=ORIENTED_EDGE('',*,*,#3893,.T.);
#4932=ORIENTED_EDGE('',*,*,#3891,.T.);
#4933=ORIENTED_EDGE('',*,*,#3894,.F.);
#4934=ORIENTED_EDGE('',*,*,#3803,.T.);
#4935=ORIENTED_EDGE('',*,*,#3895,.F.);
#4936=ORIENTED_EDGE('',*,*,#3896,.F.);
#4937=ORIENTED_EDGE('',*,*,#3897,.T.);
#4938=ORIENTED_EDGE('',*,*,#3854,.T.);
#4939=ORIENTED_EDGE('',*,*,#3898,.T.);
#4940=ORIENTED_EDGE('',*,*,#3896,.T.);
#4941=ORIENTED_EDGE('',*,*,#3899,.F.);
#4942=ORIENTED_EDGE('',*,*,#3831,.T.);
#4943=ORIENTED_EDGE('',*,*,#3900,.F.);
#4944=ORIENTED_EDGE('',*,*,#3901,.F.);
#4945=ORIENTED_EDGE('',*,*,#3902,.T.);
#4946=ORIENTED_EDGE('',*,*,#3882,.T.);
#4947=ORIENTED_EDGE('',*,*,#3903,.T.);
#4948=ORIENTED_EDGE('',*,*,#3901,.T.);
#4949=ORIENTED_EDGE('',*,*,#3904,.F.);
#4950=ORIENTED_EDGE('',*,*,#3859,.T.);
#4951=ORIENTED_EDGE('',*,*,#3905,.F.);
#4952=ORIENTED_EDGE('',*,*,#3888,.F.);
#4953=ORIENTED_EDGE('',*,*,#3906,.T.);
#4954=ORIENTED_EDGE('',*,*,#3774,.T.);
#4955=ORIENTED_EDGE('',*,*,#3778,.T.);
#4956=ORIENTED_EDGE('',*,*,#3781,.T.);
#4957=ORIENTED_EDGE('',*,*,#3784,.T.);
#4958=ORIENTED_EDGE('',*,*,#3787,.T.);
#4959=ORIENTED_EDGE('',*,*,#3790,.T.);
#4960=ORIENTED_EDGE('',*,*,#3793,.T.);
#4961=ORIENTED_EDGE('',*,*,#3796,.T.);
#4962=ORIENTED_EDGE('',*,*,#3799,.T.);
#4963=ORIENTED_EDGE('',*,*,#3889,.T.);
#4964=ORIENTED_EDGE('',*,*,#3905,.T.);
#4965=ORIENTED_EDGE('',*,*,#3858,.T.);
#4966=ORIENTED_EDGE('',*,*,#3862,.T.);
#4967=ORIENTED_EDGE('',*,*,#3865,.T.);
#4968=ORIENTED_EDGE('',*,*,#3868,.T.);
#4969=ORIENTED_EDGE('',*,*,#3871,.T.);
#4970=ORIENTED_EDGE('',*,*,#3874,.T.);
#4971=ORIENTED_EDGE('',*,*,#3877,.T.);
#4972=ORIENTED_EDGE('',*,*,#3880,.T.);
#4973=ORIENTED_EDGE('',*,*,#3883,.T.);
#4974=ORIENTED_EDGE('',*,*,#3904,.T.);
#4975=ORIENTED_EDGE('',*,*,#3900,.T.);
#4976=ORIENTED_EDGE('',*,*,#3830,.T.);
#4977=ORIENTED_EDGE('',*,*,#3834,.T.);
#4978=ORIENTED_EDGE('',*,*,#3837,.T.);
#4979=ORIENTED_EDGE('',*,*,#3840,.T.);
#4980=ORIENTED_EDGE('',*,*,#3843,.T.);
#4981=ORIENTED_EDGE('',*,*,#3846,.T.);
#4982=ORIENTED_EDGE('',*,*,#3849,.T.);
#4983=ORIENTED_EDGE('',*,*,#3852,.T.);
#4984=ORIENTED_EDGE('',*,*,#3855,.T.);
#4985=ORIENTED_EDGE('',*,*,#3899,.T.);
#4986=ORIENTED_EDGE('',*,*,#3895,.T.);
#4987=ORIENTED_EDGE('',*,*,#3802,.T.);
#4988=ORIENTED_EDGE('',*,*,#3806,.T.);
#4989=ORIENTED_EDGE('',*,*,#3809,.T.);
#4990=ORIENTED_EDGE('',*,*,#3812,.T.);
#4991=ORIENTED_EDGE('',*,*,#3815,.T.);
#4992=ORIENTED_EDGE('',*,*,#3818,.T.);
#4993=ORIENTED_EDGE('',*,*,#3821,.T.);
#4994=ORIENTED_EDGE('',*,*,#3824,.T.);
#4995=ORIENTED_EDGE('',*,*,#3827,.T.);
#4996=ORIENTED_EDGE('',*,*,#3894,.T.);
#4997=ORIENTED_EDGE('',*,*,#3890,.T.);
#4998=ORIENTED_EDGE('',*,*,#3886,.T.);
#4999=ORIENTED_EDGE('',*,*,#3772,.T.);
#5000=ORIENTED_EDGE('',*,*,#3892,.F.);
#5001=ORIENTED_EDGE('',*,*,#3893,.F.);
#5002=ORIENTED_EDGE('',*,*,#3825,.T.);
#5003=ORIENTED_EDGE('',*,*,#3822,.T.);
#5004=ORIENTED_EDGE('',*,*,#3819,.T.);
#5005=ORIENTED_EDGE('',*,*,#3816,.T.);
#5006=ORIENTED_EDGE('',*,*,#3813,.T.);
#5007=ORIENTED_EDGE('',*,*,#3810,.T.);
#5008=ORIENTED_EDGE('',*,*,#3807,.T.);
#5009=ORIENTED_EDGE('',*,*,#3804,.T.);
#5010=ORIENTED_EDGE('',*,*,#3800,.T.);
#5011=ORIENTED_EDGE('',*,*,#3897,.F.);
#5012=ORIENTED_EDGE('',*,*,#3898,.F.);
#5013=ORIENTED_EDGE('',*,*,#3853,.T.);
#5014=ORIENTED_EDGE('',*,*,#3850,.T.);
#5015=ORIENTED_EDGE('',*,*,#3847,.T.);
#5016=ORIENTED_EDGE('',*,*,#3844,.T.);
#5017=ORIENTED_EDGE('',*,*,#3841,.T.);
#5018=ORIENTED_EDGE('',*,*,#3838,.T.);
#5019=ORIENTED_EDGE('',*,*,#3835,.T.);
#5020=ORIENTED_EDGE('',*,*,#3832,.T.);
#5021=ORIENTED_EDGE('',*,*,#3828,.T.);
#5022=ORIENTED_EDGE('',*,*,#3902,.F.);
#5023=ORIENTED_EDGE('',*,*,#3903,.F.);
#5024=ORIENTED_EDGE('',*,*,#3881,.T.);
#5025=ORIENTED_EDGE('',*,*,#3878,.T.);
#5026=ORIENTED_EDGE('',*,*,#3875,.T.);
#5027=ORIENTED_EDGE('',*,*,#3872,.T.);
#5028=ORIENTED_EDGE('',*,*,#3869,.T.);
#5029=ORIENTED_EDGE('',*,*,#3866,.T.);
#5030=ORIENTED_EDGE('',*,*,#3863,.T.);
#5031=ORIENTED_EDGE('',*,*,#3860,.T.);
#5032=ORIENTED_EDGE('',*,*,#3856,.T.);
#5033=ORIENTED_EDGE('',*,*,#3906,.F.);
#5034=ORIENTED_EDGE('',*,*,#3887,.F.);
#5035=ORIENTED_EDGE('',*,*,#3797,.T.);
#5036=ORIENTED_EDGE('',*,*,#3794,.T.);
#5037=ORIENTED_EDGE('',*,*,#3791,.T.);
#5038=ORIENTED_EDGE('',*,*,#3788,.T.);
#5039=ORIENTED_EDGE('',*,*,#3785,.T.);
#5040=ORIENTED_EDGE('',*,*,#3782,.T.);
#5041=ORIENTED_EDGE('',*,*,#3779,.T.);
#5042=ORIENTED_EDGE('',*,*,#3776,.T.);
#5043=ORIENTED_EDGE('',*,*,#3884,.T.);
#5932=CYLINDRICAL_SURFACE('',#6955,0.21);
#6084=ADVANCED_FACE('',(#1021),#741,.F.);
#6085=ADVANCED_FACE('',(#1022),#742,.F.);
#6086=ADVANCED_FACE('',(#1023),#743,.F.);
#6087=ADVANCED_FACE('',(#1024),#744,.F.);
#6088=ADVANCED_FACE('',(#1025),#745,.F.);
#6089=ADVANCED_FACE('',(#1026),#746,.F.);
#6090=ADVANCED_FACE('',(#1027),#747,.F.);
#6091=ADVANCED_FACE('',(#1028),#748,.F.);
#6092=ADVANCED_FACE('',(#1029),#749,.F.);
#6093=ADVANCED_FACE('',(#1030),#750,.F.);
#6094=ADVANCED_FACE('',(#1031),#751,.F.);
#6095=ADVANCED_FACE('',(#1032),#752,.F.);
#6096=ADVANCED_FACE('',(#1033),#753,.F.);
#6097=ADVANCED_FACE('',(#1034),#754,.F.);
#6098=ADVANCED_FACE('',(#1035),#755,.F.);
#6099=ADVANCED_FACE('',(#1036),#756,.F.);
#6100=ADVANCED_FACE('',(#1037),#757,.F.);
#6101=ADVANCED_FACE('',(#1038),#758,.F.);
#6102=ADVANCED_FACE('',(#1039),#759,.F.);
#6103=ADVANCED_FACE('',(#1040),#760,.F.);
#6104=ADVANCED_FACE('',(#1041),#761,.F.);
#6105=ADVANCED_FACE('',(#1042),#762,.F.);
#6106=ADVANCED_FACE('',(#1043),#763,.F.);
#6107=ADVANCED_FACE('',(#1044),#764,.F.);
#6108=ADVANCED_FACE('',(#1045),#765,.F.);
#6109=ADVANCED_FACE('',(#1046),#766,.F.);
#6110=ADVANCED_FACE('',(#1047),#767,.F.);
#6111=ADVANCED_FACE('',(#1048),#768,.F.);
#6112=ADVANCED_FACE('',(#1049),#769,.F.);
#6113=ADVANCED_FACE('',(#1050),#770,.F.);
#6114=ADVANCED_FACE('',(#1051),#771,.F.);
#6115=ADVANCED_FACE('',(#1052),#772,.F.);
#6116=ADVANCED_FACE('',(#1053),#773,.F.);
#6117=ADVANCED_FACE('',(#1054),#774,.F.);
#6118=ADVANCED_FACE('',(#1055),#775,.F.);
#6119=ADVANCED_FACE('',(#1056),#776,.F.);
#6120=ADVANCED_FACE('',(#1057),#5932,.F.);
#6121=ADVANCED_FACE('',(#1058),#777,.T.);
#6122=ADVANCED_FACE('',(#1059),#778,.T.);
#6123=ADVANCED_FACE('',(#1060),#779,.T.);
#6124=ADVANCED_FACE('',(#1061),#780,.T.);
#6125=ADVANCED_FACE('',(#1062),#781,.T.);
#6126=ADVANCED_FACE('',(#1063),#782,.T.);
#6127=ADVANCED_FACE('',(#1064),#783,.T.);
#6128=ADVANCED_FACE('',(#1065),#784,.T.);
#6129=ADVANCED_FACE('',(#1066,#610),#785,.T.);
#6130=ADVANCED_FACE('',(#1067,#611),#786,.F.);
#6339=CLOSED_SHELL('',(#6084,#6085,#6086,#6087,#6088,#6089,#6090,#6091,
#6092,#6093,#6094,#6095,#6096,#6097,#6098,#6099,#6100,#6101,#6102,#6103,
#6104,#6105,#6106,#6107,#6108,#6109,#6110,#6111,#6112,#6113,#6114,#6115,
#6116,#6117,#6118,#6119,#6120,#6121,#6122,#6123,#6124,#6125,#6126,#6127,
#6128,#6129,#6130));
#6918=AXIS2_PLACEMENT_3D('',#9725,#7919,#7920);
#6919=AXIS2_PLACEMENT_3D('',#9726,#7921,#7922);
#6920=AXIS2_PLACEMENT_3D('',#9735,#7927,#7928);
#6921=AXIS2_PLACEMENT_3D('',#9741,#7932,#7933);
#6922=AXIS2_PLACEMENT_3D('',#9747,#7937,#7938);
#6923=AXIS2_PLACEMENT_3D('',#9753,#7942,#7943);
#6924=AXIS2_PLACEMENT_3D('',#9759,#7947,#7948);
#6925=AXIS2_PLACEMENT_3D('',#9765,#7952,#7953);
#6926=AXIS2_PLACEMENT_3D('',#9771,#7957,#7958);
#6927=AXIS2_PLACEMENT_3D('',#9777,#7962,#7963);
#6928=AXIS2_PLACEMENT_3D('',#9783,#7967,#7968);
#6929=AXIS2_PLACEMENT_3D('',#9792,#7973,#7974);
#6930=AXIS2_PLACEMENT_3D('',#9798,#7978,#7979);
#6931=AXIS2_PLACEMENT_3D('',#9804,#7983,#7984);
#6932=AXIS2_PLACEMENT_3D('',#9810,#7988,#7989);
#6933=AXIS2_PLACEMENT_3D('',#9816,#7993,#7994);
#6934=AXIS2_PLACEMENT_3D('',#9822,#7998,#7999);
#6935=AXIS2_PLACEMENT_3D('',#9828,#8003,#8004);
#6936=AXIS2_PLACEMENT_3D('',#9834,#8008,#8009);
#6937=AXIS2_PLACEMENT_3D('',#9840,#8013,#8014);
#6938=AXIS2_PLACEMENT_3D('',#9849,#8019,#8020);
#6939=AXIS2_PLACEMENT_3D('',#9855,#8024,#8025);
#6940=AXIS2_PLACEMENT_3D('',#9861,#8029,#8030);
#6941=AXIS2_PLACEMENT_3D('',#9867,#8034,#8035);
#6942=AXIS2_PLACEMENT_3D('',#9873,#8039,#8040);
#6943=AXIS2_PLACEMENT_3D('',#9879,#8044,#8045);
#6944=AXIS2_PLACEMENT_3D('',#9885,#8049,#8050);
#6945=AXIS2_PLACEMENT_3D('',#9891,#8054,#8055);
#6946=AXIS2_PLACEMENT_3D('',#9897,#8059,#8060);
#6947=AXIS2_PLACEMENT_3D('',#9906,#8065,#8066);
#6948=AXIS2_PLACEMENT_3D('',#9912,#8070,#8071);
#6949=AXIS2_PLACEMENT_3D('',#9918,#8075,#8076);
#6950=AXIS2_PLACEMENT_3D('',#9924,#8080,#8081);
#6951=AXIS2_PLACEMENT_3D('',#9930,#8085,#8086);
#6952=AXIS2_PLACEMENT_3D('',#9936,#8090,#8091);
#6953=AXIS2_PLACEMENT_3D('',#9942,#8095,#8096);
#6954=AXIS2_PLACEMENT_3D('',#9948,#8100,#8101);
#6955=AXIS2_PLACEMENT_3D('',#9954,#8105,#8106);
#6956=AXIS2_PLACEMENT_3D('',#9956,#8107,#8108);
#6957=AXIS2_PLACEMENT_3D('',#9959,#8110,#8111);
#6958=AXIS2_PLACEMENT_3D('',#9960,#8112,#8113);
#6959=AXIS2_PLACEMENT_3D('',#9966,#8117,#8118);
#6960=AXIS2_PLACEMENT_3D('',#9972,#8122,#8123);
#6961=AXIS2_PLACEMENT_3D('',#9975,#8126,#8127);
#6962=AXIS2_PLACEMENT_3D('',#9981,#8131,#8132);
#6963=AXIS2_PLACEMENT_3D('',#9984,#8135,#8136);
#6964=AXIS2_PLACEMENT_3D('',#9990,#8140,#8141);
#6965=AXIS2_PLACEMENT_3D('',#9993,#8144,#8145);
#6966=AXIS2_PLACEMENT_3D('',#9996,#8148,#8149);
#6967=AXIS2_PLACEMENT_3D('',#9997,#8150,#8151);
#7919=DIRECTION('axis',(0.,0.,1.));
#7920=DIRECTION('refdir',(1.,0.,0.));
#7921=DIRECTION('center_axis',(0.,0.,-1.));
#7922=DIRECTION('ref_axis',(0.,1.,0.));
#7923=DIRECTION('',(0.,1.,0.));
#7924=DIRECTION('',(1.,0.,0.));
#7925=DIRECTION('',(0.,-1.,0.));
#7926=DIRECTION('',(1.,0.,0.));
#7927=DIRECTION('center_axis',(0.,1.,-8.88178419700125E-16));
#7928=DIRECTION('ref_axis',(0.,8.88178419700125E-16,1.));
#7929=DIRECTION('',(0.,8.88178419700125E-16,1.));
#7930=DIRECTION('',(1.,0.,0.));
#7931=DIRECTION('',(0.,-8.88178419700125E-16,-1.));
#7932=DIRECTION('center_axis',(0.,-7.40148683083439E-16,-1.));
#7933=DIRECTION('ref_axis',(0.,1.,-7.40148683083439E-16));
#7934=DIRECTION('',(0.,1.,-7.40148683083439E-16));
#7935=DIRECTION('',(1.,0.,0.));
#7936=DIRECTION('',(0.,-1.,7.40148683083439E-16));
#7937=DIRECTION('center_axis',(0.,-0.707106781186547,-0.707106781186548));
#7938=DIRECTION('ref_axis',(0.,0.707106781186548,-0.707106781186547));
#7939=DIRECTION('',(0.,0.707106781186548,-0.707106781186547));
#7940=DIRECTION('',(1.,0.,0.));
#7941=DIRECTION('',(0.,-0.707106781186548,0.707106781186547));
#7942=DIRECTION('center_axis',(0.,-1.,2.77555756156289E-16));
#7943=DIRECTION('ref_axis',(0.,-2.77555756156289E-16,-1.));
#7944=DIRECTION('',(0.,-2.77555756156289E-16,-1.));
#7945=DIRECTION('',(1.,0.,0.));
#7946=DIRECTION('',(0.,2.77555756156289E-16,1.));
#7947=DIRECTION('center_axis',(0.,-0.707106781186547,0.707106781186548));
#7948=DIRECTION('ref_axis',(0.,-0.707106781186548,-0.707106781186547));
#7949=DIRECTION('',(0.,-0.707106781186548,-0.707106781186547));
#7950=DIRECTION('',(1.,0.,0.));
#7951=DIRECTION('',(0.,0.707106781186548,0.707106781186547));
#7952=DIRECTION('center_axis',(0.,7.40148683083438E-16,1.));
#7953=DIRECTION('ref_axis',(0.,-1.,7.40148683083438E-16));
#7954=DIRECTION('',(0.,-1.,7.40148683083438E-16));
#7955=DIRECTION('',(1.,0.,0.));
#7956=DIRECTION('',(0.,1.,-7.40148683083438E-16));
#7957=DIRECTION('center_axis',(0.,1.,-4.44089209850063E-16));
#7958=DIRECTION('ref_axis',(0.,4.44089209850063E-16,1.));
#7959=DIRECTION('',(0.,4.44089209850063E-16,1.));
#7960=DIRECTION('',(1.,0.,0.));
#7961=DIRECTION('',(0.,-4.44089209850063E-16,-1.));
#7962=DIRECTION('center_axis',(0.,2.41352831440251E-16,1.));
#7963=DIRECTION('ref_axis',(0.,-1.,2.41352831440251E-16));
#7964=DIRECTION('',(0.,-1.,2.41352831440251E-16));
#7965=DIRECTION('',(-1.,0.,0.));
#7966=DIRECTION('',(0.,1.,-2.41352831440251E-16));
#7967=DIRECTION('center_axis',(0.,-1.,2.41352831440251E-16));
#7968=DIRECTION('ref_axis',(0.,-2.41352831440251E-16,-1.));
#7969=DIRECTION('',(0.,-2.41352831440251E-16,-1.));
#7970=DIRECTION('',(1.,0.,0.));
#7971=DIRECTION('',(0.,2.41352831440251E-16,1.));
#7972=DIRECTION('',(1.,0.,0.));
#7973=DIRECTION('center_axis',(0.,0.,-1.));
#7974=DIRECTION('ref_axis',(0.,1.,0.));
#7975=DIRECTION('',(0.,1.,0.));
#7976=DIRECTION('',(1.,0.,0.));
#7977=DIRECTION('',(0.,-1.,0.));
#7978=DIRECTION('center_axis',(0.,-1.,0.));
#7979=DIRECTION('ref_axis',(0.,0.,-1.));
#7980=DIRECTION('',(0.,0.,-1.));
#7981=DIRECTION('',(1.,0.,0.));
#7982=DIRECTION('',(0.,0.,1.));
#7983=DIRECTION('center_axis',(0.,-0.707106781186547,0.707106781186548));
#7984=DIRECTION('ref_axis',(0.,-0.707106781186548,-0.707106781186547));
#7985=DIRECTION('',(0.,-0.707106781186548,-0.707106781186547));
#7986=DIRECTION('',(1.,0.,0.));
#7987=DIRECTION('',(0.,0.707106781186548,0.707106781186547));
#7988=DIRECTION('center_axis',(0.,0.,1.));
#7989=DIRECTION('ref_axis',(0.,-1.,0.));
#7990=DIRECTION('',(0.,-1.,0.));
#7991=DIRECTION('',(1.,0.,0.));
#7992=DIRECTION('',(0.,1.,0.));
#7993=DIRECTION('center_axis',(0.,0.707106781186548,0.707106781186547));
#7994=DIRECTION('ref_axis',(0.,-0.707106781186547,0.707106781186548));
#7995=DIRECTION('',(0.,-0.707106781186547,0.707106781186548));
#7996=DIRECTION('',(1.,0.,0.));
#7997=DIRECTION('',(0.,0.707106781186547,-0.707106781186548));
#7998=DIRECTION('center_axis',(0.,1.,0.));
#7999=DIRECTION('ref_axis',(0.,0.,1.));
#8000=DIRECTION('',(0.,0.,1.));
#8001=DIRECTION('',(1.,0.,0.));
#8002=DIRECTION('',(0.,0.,-1.));
#8003=DIRECTION('center_axis',(0.,0.,-1.));
#8004=DIRECTION('ref_axis',(0.,1.,0.));
#8005=DIRECTION('',(0.,1.,0.));
#8006=DIRECTION('',(1.,0.,0.));
#8007=DIRECTION('',(0.,-1.,0.));
#8008=DIRECTION('center_axis',(0.,1.,-2.41352831440251E-16));
#8009=DIRECTION('ref_axis',(0.,2.41352831440251E-16,1.));
#8010=DIRECTION('',(0.,2.41352831440251E-16,1.));
#8011=DIRECTION('',(-1.,0.,0.));
#8012=DIRECTION('',(0.,-2.41352831440251E-16,-1.));
#8013=DIRECTION('center_axis',(0.,0.,1.));
#8014=DIRECTION('ref_axis',(0.,-1.,0.));
#8015=DIRECTION('',(0.,-1.,0.));
#8016=DIRECTION('',(1.,0.,0.));
#8017=DIRECTION('',(0.,1.,0.));
#8018=DIRECTION('',(1.,0.,0.));
#8019=DIRECTION('center_axis',(0.,-1.,0.));
#8020=DIRECTION('ref_axis',(0.,0.,-1.));
#8021=DIRECTION('',(0.,0.,-1.));
#8022=DIRECTION('',(1.,0.,0.));
#8023=DIRECTION('',(0.,0.,1.));
#8024=DIRECTION('center_axis',(0.,0.,1.));
#8025=DIRECTION('ref_axis',(0.,-1.,0.));
#8026=DIRECTION('',(0.,-1.,0.));
#8027=DIRECTION('',(1.,0.,0.));
#8028=DIRECTION('',(0.,1.,0.));
#8029=DIRECTION('center_axis',(0.,0.707106781186548,0.707106781186548));
#8030=DIRECTION('ref_axis',(0.,-0.707106781186548,0.707106781186548));
#8031=DIRECTION('',(0.,-0.707106781186548,0.707106781186548));
#8032=DIRECTION('',(1.,0.,0.));
#8033=DIRECTION('',(0.,0.707106781186548,-0.707106781186548));
#8034=DIRECTION('center_axis',(0.,1.,0.));
#8035=DIRECTION('ref_axis',(0.,0.,1.));
#8036=DIRECTION('',(0.,0.,1.));
#8037=DIRECTION('',(1.,0.,0.));
#8038=DIRECTION('',(0.,0.,-1.));
#8039=DIRECTION('center_axis',(0.,0.707106781186548,-0.707106781186547));
#8040=DIRECTION('ref_axis',(0.,0.707106781186547,0.707106781186548));
#8041=DIRECTION('',(0.,0.707106781186547,0.707106781186548));
#8042=DIRECTION('',(1.,0.,0.));
#8043=DIRECTION('',(0.,-0.707106781186547,-0.707106781186548));
#8044=DIRECTION('center_axis',(0.,-7.40148683083438E-16,-1.));
#8045=DIRECTION('ref_axis',(0.,1.,-7.40148683083438E-16));
#8046=DIRECTION('',(0.,1.,-7.40148683083438E-16));
#8047=DIRECTION('',(1.,0.,0.));
#8048=DIRECTION('',(0.,-1.,7.40148683083438E-16));
#8049=DIRECTION('center_axis',(0.,-1.,0.));
#8050=DIRECTION('ref_axis',(0.,0.,-1.));
#8051=DIRECTION('',(0.,0.,-1.));
#8052=DIRECTION('',(1.,0.,0.));
#8053=DIRECTION('',(0.,0.,1.));
#8054=DIRECTION('center_axis',(0.,0.,-1.));
#8055=DIRECTION('ref_axis',(0.,1.,0.));
#8056=DIRECTION('',(0.,1.,0.));
#8057=DIRECTION('',(-1.,0.,0.));
#8058=DIRECTION('',(0.,-1.,0.));
#8059=DIRECTION('center_axis',(0.,1.,0.));
#8060=DIRECTION('ref_axis',(0.,0.,1.));
#8061=DIRECTION('',(0.,0.,1.));
#8062=DIRECTION('',(1.,0.,0.));
#8063=DIRECTION('',(0.,0.,-1.));
#8064=DIRECTION('',(1.,0.,0.));
#8065=DIRECTION('center_axis',(0.,0.,1.));
#8066=DIRECTION('ref_axis',(0.,-1.,0.));
#8067=DIRECTION('',(0.,-1.,0.));
#8068=DIRECTION('',(1.,0.,0.));
#8069=DIRECTION('',(0.,1.,0.));
#8070=DIRECTION('center_axis',(0.,1.,0.));
#8071=DIRECTION('ref_axis',(0.,0.,1.));
#8072=DIRECTION('',(0.,0.,1.));
#8073=DIRECTION('',(1.,0.,0.));
#8074=DIRECTION('',(0.,0.,-1.));
#8075=DIRECTION('center_axis',(0.,0.707106781186547,-0.707106781186548));
#8076=DIRECTION('ref_axis',(0.,0.707106781186548,0.707106781186547));
#8077=DIRECTION('',(0.,0.707106781186548,0.707106781186547));
#8078=DIRECTION('',(1.,0.,0.));
#8079=DIRECTION('',(0.,-0.707106781186548,-0.707106781186547));
#8080=DIRECTION('center_axis',(0.,0.,-1.));
#8081=DIRECTION('ref_axis',(0.,1.,0.));
#8082=DIRECTION('',(0.,1.,0.));
#8083=DIRECTION('',(1.,0.,0.));
#8084=DIRECTION('',(0.,-1.,0.));
#8085=DIRECTION('center_axis',(0.,-0.707106781186547,-0.707106781186548));
#8086=DIRECTION('ref_axis',(0.,0.707106781186548,-0.707106781186547));
#8087=DIRECTION('',(0.,0.707106781186548,-0.707106781186547));
#8088=DIRECTION('',(1.,0.,0.));
#8089=DIRECTION('',(0.,-0.707106781186548,0.707106781186547));
#8090=DIRECTION('center_axis',(0.,-1.,0.));
#8091=DIRECTION('ref_axis',(0.,0.,-1.));
#8092=DIRECTION('',(0.,0.,-1.));
#8093=DIRECTION('',(1.,0.,0.));
#8094=DIRECTION('',(0.,0.,1.));
#8095=DIRECTION('center_axis',(0.,0.,1.));
#8096=DIRECTION('ref_axis',(0.,-1.,0.));
#8097=DIRECTION('',(0.,-1.,0.));
#8098=DIRECTION('',(1.,0.,0.));
#8099=DIRECTION('',(0.,1.,0.));
#8100=DIRECTION('center_axis',(0.,-1.,0.));
#8101=DIRECTION('ref_axis',(0.,0.,-1.));
#8102=DIRECTION('',(0.,0.,-1.));
#8103=DIRECTION('',(-1.,0.,0.));
#8104=DIRECTION('',(0.,0.,1.));
#8105=DIRECTION('center_axis',(1.,0.,0.));
#8106=DIRECTION('ref_axis',(0.,0.,-1.));
#8107=DIRECTION('center_axis',(1.,0.,0.));
#8108=DIRECTION('ref_axis',(0.,0.,-1.));
#8109=DIRECTION('',(1.,0.,0.));
#8110=DIRECTION('center_axis',(-1.,0.,0.));
#8111=DIRECTION('ref_axis',(0.,0.,-1.));
#8112=DIRECTION('center_axis',(0.,1.,0.));
#8113=DIRECTION('ref_axis',(0.,0.,1.));
#8114=DIRECTION('',(0.,0.,1.));
#8115=DIRECTION('',(1.,0.,0.));
#8116=DIRECTION('',(0.,0.,1.));
#8117=DIRECTION('center_axis',(0.,1.,0.));
#8118=DIRECTION('ref_axis',(0.,0.,1.));
#8119=DIRECTION('',(0.,0.,1.));
#8120=DIRECTION('',(1.,0.,0.));
#8121=DIRECTION('',(0.,0.,1.));
#8122=DIRECTION('center_axis',(0.,0.,-1.));
#8123=DIRECTION('ref_axis',(0.,1.,0.));
#8124=DIRECTION('',(0.,1.,0.));
#8125=DIRECTION('',(0.,1.,0.));
#8126=DIRECTION('center_axis',(0.,0.,-1.));
#8127=DIRECTION('ref_axis',(0.,1.,0.));
#8128=DIRECTION('',(0.,1.,0.));
#8129=DIRECTION('',(1.,0.,0.));
#8130=DIRECTION('',(0.,1.,0.));
#8131=DIRECTION('center_axis',(0.,-1.,0.));
#8132=DIRECTION('ref_axis',(0.,0.,-1.));
#8133=DIRECTION('',(0.,0.,-1.));
#8134=DIRECTION('',(0.,0.,-1.));
#8135=DIRECTION('center_axis',(0.,-1.,0.));
#8136=DIRECTION('ref_axis',(0.,0.,-1.));
#8137=DIRECTION('',(0.,0.,-1.));
#8138=DIRECTION('',(1.,0.,0.));
#8139=DIRECTION('',(0.,0.,-1.));
#8140=DIRECTION('center_axis',(0.,0.,1.));
#8141=DIRECTION('ref_axis',(0.,-1.,0.));
#8142=DIRECTION('',(0.,-1.,0.));
#8143=DIRECTION('',(0.,-1.,0.));
#8144=DIRECTION('center_axis',(0.,0.,1.));
#8145=DIRECTION('ref_axis',(0.,-1.,0.));
#8146=DIRECTION('',(0.,-1.,0.));
#8147=DIRECTION('',(0.,-1.,0.));
#8148=DIRECTION('center_axis',(1.,0.,0.));
#8149=DIRECTION('ref_axis',(0.,0.,-1.));
#8150=DIRECTION('center_axis',(1.,0.,0.));
#8151=DIRECTION('ref_axis',(0.,0.,-1.));
#9725=CARTESIAN_POINT('',(0.,0.,0.));
#9726=CARTESIAN_POINT('Origin',(-0.1,0.82,-0.3));
#9727=CARTESIAN_POINT('',(0.,0.82,-0.3));
#9728=CARTESIAN_POINT('',(0.,1.,-0.3));
#9729=CARTESIAN_POINT('',(0.,0.41,-0.3));
#9730=CARTESIAN_POINT('',(20.,0.82,-0.3));
#9731=CARTESIAN_POINT('',(-0.1,0.82,-0.3));
#9732=CARTESIAN_POINT('',(20.,1.,-0.3));
#9733=CARTESIAN_POINT('',(20.,0.41,-0.3));
#9734=CARTESIAN_POINT('',(-0.05,1.,-0.3));
#9735=CARTESIAN_POINT('Origin',(-0.1,0.82,-0.55));
#9736=CARTESIAN_POINT('',(0.,0.82,-0.55));
#9737=CARTESIAN_POINT('',(0.,0.82,-0.275));
#9738=CARTESIAN_POINT('',(20.,0.82,-0.55));
#9739=CARTESIAN_POINT('',(-0.1,0.82,-0.55));
#9740=CARTESIAN_POINT('',(20.,0.82,-0.275));
#9741=CARTESIAN_POINT('Origin',(-0.1,0.67,-0.55));
#9742=CARTESIAN_POINT('',(0.,0.67,-0.55));
#9743=CARTESIAN_POINT('',(0.,0.335,-0.55));
#9744=CARTESIAN_POINT('',(20.,0.67,-0.55));
#9745=CARTESIAN_POINT('',(-0.1,0.67,-0.55));
#9746=CARTESIAN_POINT('',(20.,0.335,-0.55));
#9747=CARTESIAN_POINT('Origin',(-0.1,0.42,-0.3));
#9748=CARTESIAN_POINT('',(0.,0.42,-0.3));
#9749=CARTESIAN_POINT('',(0.,0.24,-0.12));
#9750=CARTESIAN_POINT('',(20.,0.42,-0.3));
#9751=CARTESIAN_POINT('',(-0.1,0.42,-0.3));
#9752=CARTESIAN_POINT('',(20.,0.24,-0.12));
#9753=CARTESIAN_POINT('Origin',(-0.1,0.42,0.3));
#9754=CARTESIAN_POINT('',(0.,0.42,0.3));
#9755=CARTESIAN_POINT('',(0.,0.42,0.15));
#9756=CARTESIAN_POINT('',(20.,0.42,0.3));
#9757=CARTESIAN_POINT('',(-0.1,0.42,0.3));
#9758=CARTESIAN_POINT('',(20.,0.42,0.15));
#9759=CARTESIAN_POINT('Origin',(-0.1,0.67,0.55));
#9760=CARTESIAN_POINT('',(0.,0.67,0.55));
#9761=CARTESIAN_POINT('',(6.93889390390723E-18,0.365,0.245));
#9762=CARTESIAN_POINT('',(20.,0.67,0.55));
#9763=CARTESIAN_POINT('',(-0.1,0.67,0.55));
#9764=CARTESIAN_POINT('',(20.,0.365,0.245));
#9765=CARTESIAN_POINT('Origin',(-0.1,0.82,0.55));
#9766=CARTESIAN_POINT('',(0.,0.82,0.55));
#9767=CARTESIAN_POINT('',(0.,0.41,0.55));
#9768=CARTESIAN_POINT('',(20.,0.82,0.55));
#9769=CARTESIAN_POINT('',(-0.1,0.82,0.55));
#9770=CARTESIAN_POINT('',(20.,0.41,0.55));
#9771=CARTESIAN_POINT('Origin',(-0.1,0.82,0.3));
#9772=CARTESIAN_POINT('',(0.,0.82,0.3));
#9773=CARTESIAN_POINT('',(0.,0.82,0.15));
#9774=CARTESIAN_POINT('',(20.,0.82,0.3));
#9775=CARTESIAN_POINT('',(-0.1,0.82,0.3));
#9776=CARTESIAN_POINT('',(20.,0.82,0.15));
#9777=CARTESIAN_POINT('Origin',(-0.1,1.05,0.3));
#9778=CARTESIAN_POINT('',(0.,1.,0.3));
#9779=CARTESIAN_POINT('',(0.,0.525,0.3));
#9780=CARTESIAN_POINT('',(20.,1.,0.3));
#9781=CARTESIAN_POINT('',(-0.05,1.,0.3));
#9782=CARTESIAN_POINT('',(20.,0.525,0.3));
#9783=CARTESIAN_POINT('Origin',(-0.1,-0.3,-0.82));
#9784=CARTESIAN_POINT('',(0.,-0.3,-0.82));
#9785=CARTESIAN_POINT('',(0.,-0.3,-1.));
#9786=CARTESIAN_POINT('',(0.,-0.3,-0.41));
#9787=CARTESIAN_POINT('',(20.,-0.3,-0.82));
#9788=CARTESIAN_POINT('',(-0.1,-0.3,-0.82));
#9789=CARTESIAN_POINT('',(20.,-0.3,-1.));
#9790=CARTESIAN_POINT('',(20.,-0.3,-0.41));
#9791=CARTESIAN_POINT('',(-0.05,-0.3,-1.));
#9792=CARTESIAN_POINT('Origin',(-0.1,-0.55,-0.82));
#9793=CARTESIAN_POINT('',(0.,-0.55,-0.82));
#9794=CARTESIAN_POINT('',(0.,-0.275,-0.82));
#9795=CARTESIAN_POINT('',(20.,-0.55,-0.82));
#9796=CARTESIAN_POINT('',(-0.1,-0.55,-0.82));
#9797=CARTESIAN_POINT('',(20.,-0.275,-0.82));
#9798=CARTESIAN_POINT('Origin',(-0.1,-0.55,-0.67));
#9799=CARTESIAN_POINT('',(0.,-0.55,-0.67));
#9800=CARTESIAN_POINT('',(0.,-0.55,-0.335));
#9801=CARTESIAN_POINT('',(20.,-0.55,-0.67));
#9802=CARTESIAN_POINT('',(-0.1,-0.55,-0.67));
#9803=CARTESIAN_POINT('',(20.,-0.55,-0.335));
#9804=CARTESIAN_POINT('Origin',(-0.1,-0.3,-0.42));
#9805=CARTESIAN_POINT('',(0.,-0.3,-0.42));
#9806=CARTESIAN_POINT('',(0.,-0.12,-0.24));
#9807=CARTESIAN_POINT('',(20.,-0.3,-0.42));
#9808=CARTESIAN_POINT('',(-0.1,-0.3,-0.42));
#9809=CARTESIAN_POINT('',(20.,-0.12,-0.24));
#9810=CARTESIAN_POINT('Origin',(-0.1,0.3,-0.42));
#9811=CARTESIAN_POINT('',(0.,0.3,-0.42));
#9812=CARTESIAN_POINT('',(0.,0.15,-0.42));
#9813=CARTESIAN_POINT('',(20.,0.3,-0.42));
#9814=CARTESIAN_POINT('',(-0.1,0.3,-0.42));
#9815=CARTESIAN_POINT('',(20.,0.15,-0.42));
#9816=CARTESIAN_POINT('Origin',(-0.1,0.55,-0.67));
#9817=CARTESIAN_POINT('',(0.,0.55,-0.67));
#9818=CARTESIAN_POINT('',(0.,0.245,-0.365));
#9819=CARTESIAN_POINT('',(20.,0.55,-0.67));
#9820=CARTESIAN_POINT('',(-0.1,0.55,-0.67));
#9821=CARTESIAN_POINT('',(20.,0.245,-0.365));
#9822=CARTESIAN_POINT('Origin',(-0.1,0.55,-0.82));
#9823=CARTESIAN_POINT('',(0.,0.55,-0.82));
#9824=CARTESIAN_POINT('',(0.,0.55,-0.41));
#9825=CARTESIAN_POINT('',(20.,0.55,-0.82));
#9826=CARTESIAN_POINT('',(-0.1,0.55,-0.82));
#9827=CARTESIAN_POINT('',(20.,0.55,-0.41));
#9828=CARTESIAN_POINT('Origin',(-0.1,0.3,-0.82));
#9829=CARTESIAN_POINT('',(0.,0.3,-0.82));
#9830=CARTESIAN_POINT('',(0.,0.15,-0.82));
#9831=CARTESIAN_POINT('',(20.,0.3,-0.82));
#9832=CARTESIAN_POINT('',(-0.1,0.3,-0.82));
#9833=CARTESIAN_POINT('',(20.,0.15,-0.82));
#9834=CARTESIAN_POINT('Origin',(-0.1,0.3,-1.05));
#9835=CARTESIAN_POINT('',(0.,0.3,-1.));
#9836=CARTESIAN_POINT('',(0.,0.3,-0.525));
#9837=CARTESIAN_POINT('',(20.,0.3,-1.));
#9838=CARTESIAN_POINT('',(-0.05,0.3,-1.));
#9839=CARTESIAN_POINT('',(20.,0.3,-0.525));
#9840=CARTESIAN_POINT('Origin',(-0.1,-0.82,0.3));
#9841=CARTESIAN_POINT('',(0.,-0.82,0.3));
#9842=CARTESIAN_POINT('',(0.,-1.,0.3));
#9843=CARTESIAN_POINT('',(0.,-0.41,0.3));
#9844=CARTESIAN_POINT('',(20.,-0.82,0.3));
#9845=CARTESIAN_POINT('',(-0.1,-0.82,0.3));
#9846=CARTESIAN_POINT('',(20.,-1.,0.3));
#9847=CARTESIAN_POINT('',(20.,-0.41,0.3));
#9848=CARTESIAN_POINT('',(-0.05,-1.,0.3));
#9849=CARTESIAN_POINT('Origin',(-0.1,-0.82,0.55));
#9850=CARTESIAN_POINT('',(0.,-0.82,0.55));
#9851=CARTESIAN_POINT('',(0.,-0.82,0.275));
#9852=CARTESIAN_POINT('',(20.,-0.82,0.55));
#9853=CARTESIAN_POINT('',(-0.1,-0.82,0.55));
#9854=CARTESIAN_POINT('',(20.,-0.82,0.275));
#9855=CARTESIAN_POINT('Origin',(-0.1,-0.67,0.55));
#9856=CARTESIAN_POINT('',(0.,-0.67,0.55));
#9857=CARTESIAN_POINT('',(0.,-0.335,0.55));
#9858=CARTESIAN_POINT('',(20.,-0.67,0.55));
#9859=CARTESIAN_POINT('',(-0.1,-0.67,0.55));
#9860=CARTESIAN_POINT('',(20.,-0.335,0.55));
#9861=CARTESIAN_POINT('Origin',(-0.1,-0.42,0.3));
#9862=CARTESIAN_POINT('',(0.,-0.42,0.3));
#9863=CARTESIAN_POINT('',(-6.93889390390723E-18,-0.24,0.12));
#9864=CARTESIAN_POINT('',(20.,-0.42,0.3));
#9865=CARTESIAN_POINT('',(-0.1,-0.42,0.3));
#9866=CARTESIAN_POINT('',(20.,-0.24,0.12));
#9867=CARTESIAN_POINT('Origin',(-0.1,-0.42,-0.3));
#9868=CARTESIAN_POINT('',(0.,-0.42,-0.3));
#9869=CARTESIAN_POINT('',(0.,-0.42,-0.15));
#9870=CARTESIAN_POINT('',(20.,-0.42,-0.3));
#9871=CARTESIAN_POINT('',(-0.1,-0.42,-0.3));
#9872=CARTESIAN_POINT('',(20.,-0.42,-0.15));
#9873=CARTESIAN_POINT('Origin',(-0.1,-0.67,-0.55));
#9874=CARTESIAN_POINT('',(0.,-0.67,-0.55));
#9875=CARTESIAN_POINT('',(0.,-0.365,-0.245));
#9876=CARTESIAN_POINT('',(20.,-0.67,-0.55));
#9877=CARTESIAN_POINT('',(-0.1,-0.67,-0.55));
#9878=CARTESIAN_POINT('',(20.,-0.365,-0.245));
#9879=CARTESIAN_POINT('Origin',(-0.1,-0.82,-0.55));
#9880=CARTESIAN_POINT('',(0.,-0.82,-0.55));
#9881=CARTESIAN_POINT('',(0.,-0.41,-0.55));
#9882=CARTESIAN_POINT('',(20.,-0.82,-0.55));
#9883=CARTESIAN_POINT('',(-0.1,-0.82,-0.55));
#9884=CARTESIAN_POINT('',(20.,-0.41,-0.55));
#9885=CARTESIAN_POINT('Origin',(-0.1,-0.82,-0.3));
#9886=CARTESIAN_POINT('',(0.,-0.82,-0.3));
#9887=CARTESIAN_POINT('',(0.,-0.82,-0.15));
#9888=CARTESIAN_POINT('',(20.,-0.82,-0.3));
#9889=CARTESIAN_POINT('',(-0.1,-0.82,-0.3));
#9890=CARTESIAN_POINT('',(20.,-0.82,-0.15));
#9891=CARTESIAN_POINT('Origin',(-0.1,-1.05,-0.3));
#9892=CARTESIAN_POINT('',(0.,-1.,-0.3));
#9893=CARTESIAN_POINT('',(0.,-0.525,-0.3));
#9894=CARTESIAN_POINT('',(20.,-1.,-0.3));
#9895=CARTESIAN_POINT('',(-0.05,-1.,-0.3));
#9896=CARTESIAN_POINT('',(20.,-0.525,-0.3));
#9897=CARTESIAN_POINT('Origin',(-0.1,0.3,0.82));
#9898=CARTESIAN_POINT('',(0.,0.3,0.82));
#9899=CARTESIAN_POINT('',(0.,0.3,1.));
#9900=CARTESIAN_POINT('',(0.,0.3,0.41));
#9901=CARTESIAN_POINT('',(20.,0.3,0.82));
#9902=CARTESIAN_POINT('',(-0.1,0.3,0.82));
#9903=CARTESIAN_POINT('',(20.,0.3,1.));
#9904=CARTESIAN_POINT('',(20.,0.3,0.41));
#9905=CARTESIAN_POINT('',(-0.05,0.3,1.));
#9906=CARTESIAN_POINT('Origin',(-0.1,0.55,0.82));
#9907=CARTESIAN_POINT('',(0.,0.55,0.82));
#9908=CARTESIAN_POINT('',(0.,0.275,0.82));
#9909=CARTESIAN_POINT('',(20.,0.55,0.82));
#9910=CARTESIAN_POINT('',(-0.1,0.55,0.82));
#9911=CARTESIAN_POINT('',(20.,0.275,0.82));
#9912=CARTESIAN_POINT('Origin',(-0.1,0.55,0.67));
#9913=CARTESIAN_POINT('',(0.,0.55,0.67));
#9914=CARTESIAN_POINT('',(0.,0.55,0.335));
#9915=CARTESIAN_POINT('',(20.,0.55,0.67));
#9916=CARTESIAN_POINT('',(-0.1,0.55,0.67));
#9917=CARTESIAN_POINT('',(20.,0.55,0.335));
#9918=CARTESIAN_POINT('Origin',(-0.1,0.3,0.42));
#9919=CARTESIAN_POINT('',(0.,0.3,0.42));
#9920=CARTESIAN_POINT('',(6.93889390390723E-18,0.12,0.24));
#9921=CARTESIAN_POINT('',(20.,0.3,0.42));
#9922=CARTESIAN_POINT('',(-0.1,0.3,0.42));
#9923=CARTESIAN_POINT('',(20.,0.12,0.24));
#9924=CARTESIAN_POINT('Origin',(-0.1,-0.3,0.42));
#9925=CARTESIAN_POINT('',(0.,-0.3,0.42));
#9926=CARTESIAN_POINT('',(0.,-0.15,0.42));
#9927=CARTESIAN_POINT('',(20.,-0.3,0.42));
#9928=CARTESIAN_POINT('',(-0.1,-0.3,0.42));
#9929=CARTESIAN_POINT('',(20.,-0.15,0.42));
#9930=CARTESIAN_POINT('Origin',(-0.1,-0.55,0.67));
#9931=CARTESIAN_POINT('',(0.,-0.55,0.67));
#9932=CARTESIAN_POINT('',(6.93889390390723E-18,-0.245,0.365));
#9933=CARTESIAN_POINT('',(20.,-0.55,0.67));
#9934=CARTESIAN_POINT('',(-0.1,-0.55,0.67));
#9935=CARTESIAN_POINT('',(20.,-0.245,0.365));
#9936=CARTESIAN_POINT('Origin',(-0.1,-0.55,0.82));
#9937=CARTESIAN_POINT('',(0.,-0.55,0.82));
#9938=CARTESIAN_POINT('',(0.,-0.55,0.41));
#9939=CARTESIAN_POINT('',(20.,-0.55,0.82));
#9940=CARTESIAN_POINT('',(-0.1,-0.55,0.82));
#9941=CARTESIAN_POINT('',(20.,-0.55,0.41));
#9942=CARTESIAN_POINT('Origin',(-0.1,-0.3,0.82));
#9943=CARTESIAN_POINT('',(0.,-0.3,0.82));
#9944=CARTESIAN_POINT('',(0.,-0.15,0.82));
#9945=CARTESIAN_POINT('',(20.,-0.3,0.82));
#9946=CARTESIAN_POINT('',(-0.1,-0.3,0.82));
#9947=CARTESIAN_POINT('',(20.,-0.15,0.82));
#9948=CARTESIAN_POINT('Origin',(-0.1,-0.3,1.05));
#9949=CARTESIAN_POINT('',(0.,-0.3,1.));
#9950=CARTESIAN_POINT('',(0.,-0.3,0.525));
#9951=CARTESIAN_POINT('',(20.,-0.3,1.));
#9952=CARTESIAN_POINT('',(-0.05,-0.3,1.));
#9953=CARTESIAN_POINT('',(20.,-0.3,0.525));
#9954=CARTESIAN_POINT('Origin',(-0.1,0.,0.));
#9955=CARTESIAN_POINT('',(0.,-2.57175827820944E-17,0.21));
#9956=CARTESIAN_POINT('Origin',(0.,0.,0.));
#9957=CARTESIAN_POINT('',(20.,2.57175827820944E-17,0.21));
#9958=CARTESIAN_POINT('',(-0.1,-2.57175827820944E-17,0.21));
#9959=CARTESIAN_POINT('Origin',(20.,0.,0.));
#9960=CARTESIAN_POINT('Origin',(0.,1.,-1.));
#9961=CARTESIAN_POINT('',(0.,1.,1.));
#9962=CARTESIAN_POINT('',(0.,1.,-1.));
#9963=CARTESIAN_POINT('',(20.,1.,1.));
#9964=CARTESIAN_POINT('',(0.,1.,1.));
#9965=CARTESIAN_POINT('',(20.,1.,-1.));
#9966=CARTESIAN_POINT('Origin',(0.,1.,-1.));
#9967=CARTESIAN_POINT('',(20.,1.,-1.));
#9968=CARTESIAN_POINT('',(20.,1.,-1.));
#9969=CARTESIAN_POINT('',(0.,1.,-1.));
#9970=CARTESIAN_POINT('',(0.,1.,-1.));
#9971=CARTESIAN_POINT('',(0.,1.,-1.));
#9972=CARTESIAN_POINT('Origin',(0.,-1.,-1.));
#9973=CARTESIAN_POINT('',(0.,-1.,-1.));
#9974=CARTESIAN_POINT('',(20.,-1.,-1.));
#9975=CARTESIAN_POINT('Origin',(0.,-1.,-1.));
#9976=CARTESIAN_POINT('',(20.,-1.,-1.));
#9977=CARTESIAN_POINT('',(20.,-1.,-1.));
#9978=CARTESIAN_POINT('',(0.,-1.,-1.));
#9979=CARTESIAN_POINT('',(0.,-1.,-1.));
#9980=CARTESIAN_POINT('',(0.,-1.,-1.));
#9981=CARTESIAN_POINT('Origin',(0.,-1.,1.));
#9982=CARTESIAN_POINT('',(0.,-1.,1.));
#9983=CARTESIAN_POINT('',(20.,-1.,1.));
#9984=CARTESIAN_POINT('Origin',(0.,-1.,1.));
#9985=CARTESIAN_POINT('',(20.,-1.,1.));
#9986=CARTESIAN_POINT('',(20.,-1.,1.));
#9987=CARTESIAN_POINT('',(0.,-1.,1.));
#9988=CARTESIAN_POINT('',(0.,-1.,1.));
#9989=CARTESIAN_POINT('',(0.,-1.,1.));
#9990=CARTESIAN_POINT('Origin',(0.,1.,1.));
#9991=CARTESIAN_POINT('',(0.,1.,1.));
#9992=CARTESIAN_POINT('',(20.,1.,1.));
#9993=CARTESIAN_POINT('Origin',(0.,1.,1.));
#9994=CARTESIAN_POINT('',(20.,1.,1.));
#9995=CARTESIAN_POINT('',(0.,1.,1.));
#9996=CARTESIAN_POINT('Origin',(20.,0.,0.));
#9997=CARTESIAN_POINT('Origin',(0.,0.,0.));
#11503=UNCERTAINTY_MEASURE_WITH_UNIT(LENGTH_MEASURE(0.001),#11560,
'DISTANCE_ACCURACY_VALUE',
'Maximum model space distance between geometric entities at asserted c
onnectivities');
#11522=UNCERTAINTY_MEASURE_WITH_UNIT(LENGTH_MEASURE(0.001),#11560,
'DISTANCE_ACCURACY_VALUE',
'Maximum model space distance between geometric entities at asserted c
onnectivities');
#11540=(
GEOMETRIC_REPRESENTATION_CONTEXT(3)
GLOBAL_UNCERTAINTY_ASSIGNED_CONTEXT((#11503))
GLOBAL_UNIT_ASSIGNED_CONTEXT((#11560,#11562,#11563))
REPRESENTATION_CONTEXT('','3D')
);
#11559=(
GEOMETRIC_REPRESENTATION_CONTEXT(3)
GLOBAL_UNCERTAINTY_ASSIGNED_CONTEXT((#11522))
GLOBAL_UNIT_ASSIGNED_CONTEXT((#11560,#11562,#11563))
REPRESENTATION_CONTEXT('','3D')
);
#11560=(
LENGTH_UNIT()
NAMED_UNIT(*)
SI_UNIT(.CENTI.,.METRE.)
);
#11562=(
NAMED_UNIT(*)
PLANE_ANGLE_UNIT()
SI_UNIT($,.RADIAN.)
);
#11563=(
NAMED_UNIT(*)
SI_UNIT($,.STERADIAN.)
SOLID_ANGLE_UNIT()
);
#11581=SHAPE_DEFINITION_REPRESENTATION(#11617,#11738);
#11617=PRODUCT_DEFINITION_SHAPE('',$,#11775);
#11738=SHAPE_REPRESENTATION('',(#6918),#11540);
#11757=PRODUCT_DEFINITION_CONTEXT('part definition',#11867,'design');
#11775=PRODUCT_DEFINITION('Slotted Extrusion - 20 x 20 x 200 mm',
'Slotted Extrusion - 20 x 20 x 200 mm',#11811,#11757);
#11811=PRODUCT_DEFINITION_FORMATION('',$,#11886);
#11867=APPLICATION_CONTEXT(
'Core Data for Automotive Mechanical Design Process');
#11868=PRODUCT_CONTEXT('part definition',#11867,'mechanical');
#11886=PRODUCT('Slotted Extrusion - 20 x 20 x 200 mm',
'Slotted Extrusion - 20 x 20 x 200 mm',
'Slotted Extrusion - 20 x 20 x 200 mm',(#11868));
#11975=COLOUR_RGB('Off White',0.89,0.88,0.83);
#11976=FILL_AREA_STYLE_COLOUR('',#11975);
#11977=FILL_AREA_STYLE('',(#11976));
#11978=SURFACE_STYLE_FILL_AREA(#11977);
#11979=SURFACE_SIDE_STYLE('',(#11978));
#11980=SURFACE_STYLE_USAGE(.BOTH.,#11979);
#11981=PRESENTATION_STYLE_ASSIGNMENT((#11980));
ENDSEC;
END-ISO-10303-21;
